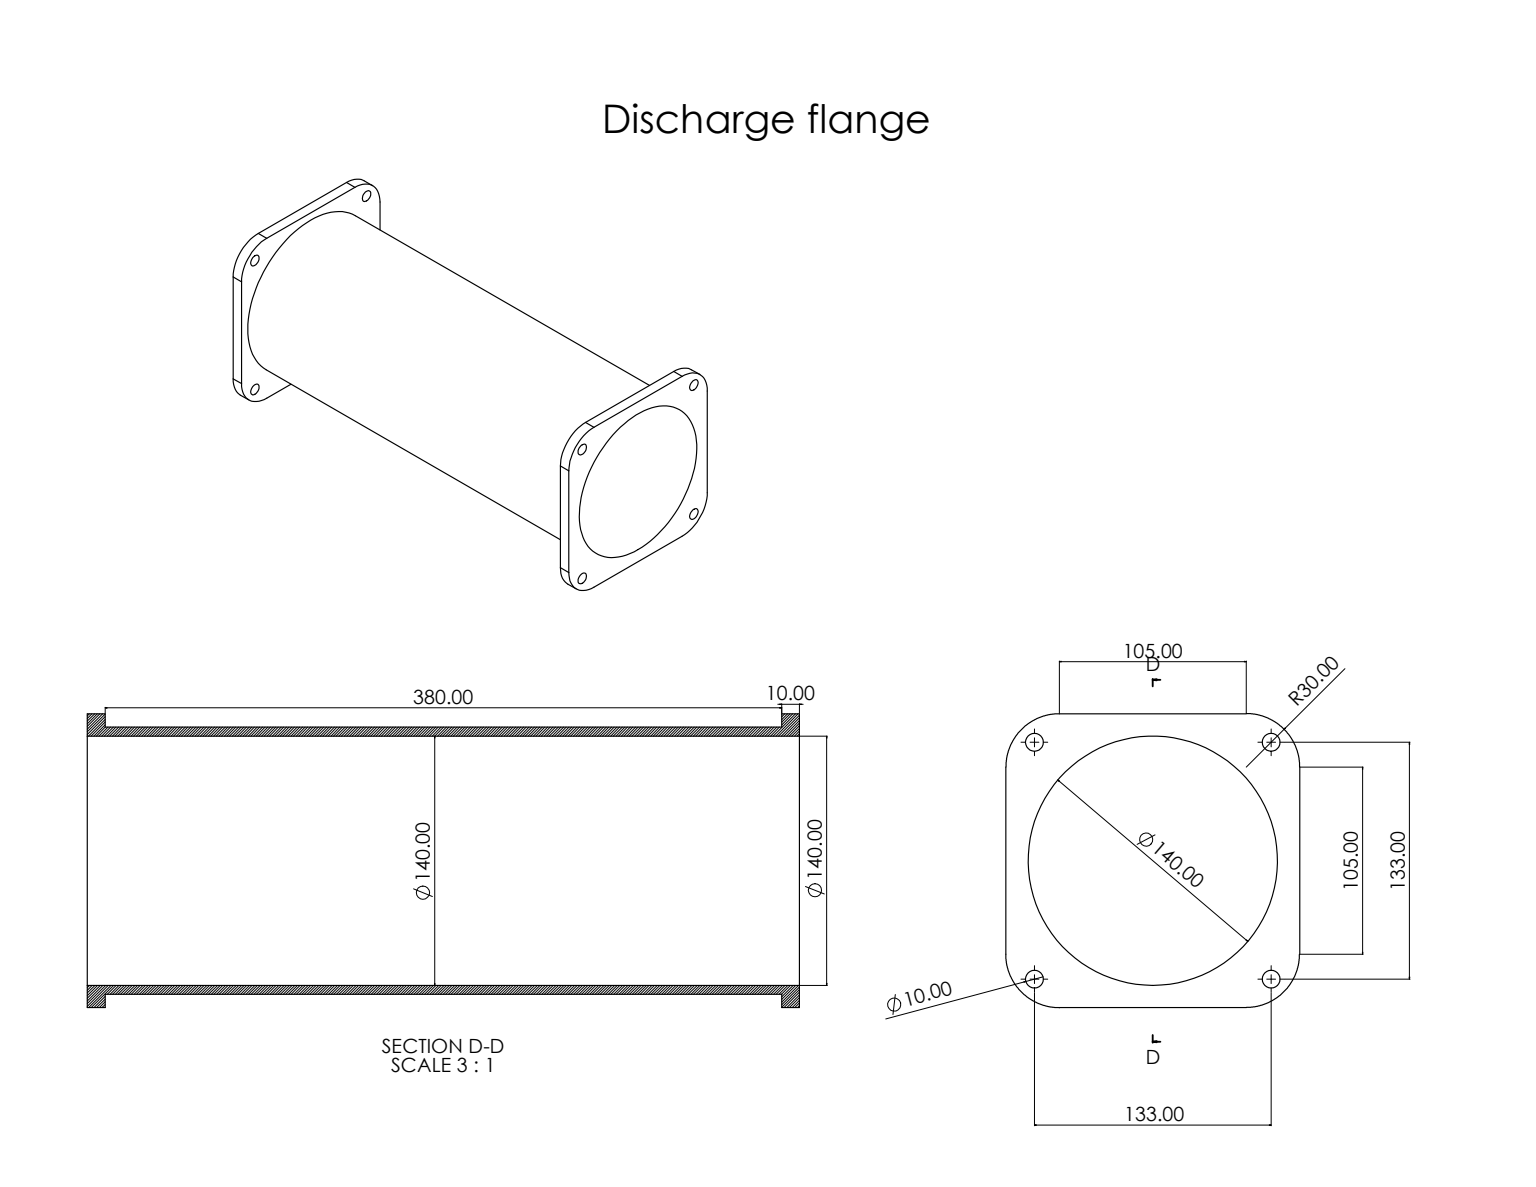
ISO-10303-21;
HEADER;
FILE_DESCRIPTION (('STEP AP214'),
    '1' );
FILE_NAME ('Discharge flange.step',
    '2026-10-27T19:20:31',
    ( '' ),
    ( '' ),
    'SwSTEP 2.0',
    'SolidWorks 2025',
    '' );
FILE_SCHEMA (( 'AUTOMOTIVE_DESIGN' ));
ENDSEC;

DATA;
#22=DIRECTION ( 'NONE',  ( 0.000000000000000000, 0.000000000000000000, 1.000000000000000000 ) ) ;
#32=CARTESIAN_POINT ( 'NONE',  ( -190.0000000000000000, 52.50000000000007816, 52.49999999999999289 ) ) ;
#50=FACE_OUTER_BOUND ( 'NONE', #10007, .T. ) ;
#60=VERTEX_POINT ( 'NONE', #18074 ) ;
#118=ORIENTED_EDGE ( 'NONE', *, *, #8682, .F. ) ;
#155=CARTESIAN_POINT ( 'NONE',  ( 190.0000000000000000, -66.50000000000001421, -66.50000000000005684 ) ) ;
#163=ORIENTED_EDGE ( 'NONE', *, *, #20627, .T. ) ;
#171=CARTESIAN_POINT ( 'NONE',  ( -200.0000000000000000, -66.50000000000001421, -66.50000000000005684 ) ) ;
#193=ADVANCED_FACE ( 'NONE', ( #5707 ), #22219, .T. ) ;
#218=VERTEX_POINT ( 'NONE', #16347 ) ;
#269=DIRECTION ( 'NONE',  ( 0.000000000000000000, -1.000000000000000000, 0.000000000000000000 ) ) ;
#281=ORIENTED_EDGE ( 'NONE', *, *, #13368, .T. ) ;
#283=CARTESIAN_POINT ( 'NONE',  ( -200.0000000000000000, 52.49999999999987210, -82.49999999999998579 ) ) ;
#287=VERTEX_POINT ( 'NONE', #6242 ) ;
#300=ADVANCED_FACE ( 'NONE', ( #8363, #8229, #20751, #2125, #20481, #18473 ), #22483, .F. ) ;
#304=ADVANCED_FACE ( 'NONE', ( #10498 ), #8499, .T. ) ;
#317=DIRECTION ( 'NONE',  ( 1.000000000000000000, -1.836970198721030181E-16, -0.000000000000000000 ) ) ;
#324=DIRECTION ( 'NONE',  ( 1.000000000000000000, 1.836970198721030181E-16, 0.000000000000000000 ) ) ;
#390=ORIENTED_EDGE ( 'NONE', *, *, #13074, .F. ) ;
#407=DIRECTION ( 'NONE',  ( 0.000000000000000000, 0.000000000000000000, 1.000000000000000000 ) ) ;
#423=AXIS2_PLACEMENT_3D ( 'NONE', #16508, #2685, #22769 ) ;
#428=EDGE_LOOP ( 'NONE', ( #390, #21002 ) ) ;
#432=EDGE_LOOP ( 'NONE', ( #11863, #1832, #6303, #14953 ) ) ;
#433=VERTEX_POINT ( 'NONE', #24106 ) ;
#441=FACE_BOUND ( 'NONE', #16176, .T. ) ;
#484=DIRECTION ( 'NONE',  ( -1.000000000000000000, -1.836970198721030181E-16, -0.000000000000000000 ) ) ;
#497=AXIS2_PLACEMENT_3D ( 'NONE', #8550, #23068, #15061 ) ;
#509=VECTOR ( 'NONE', #21184, 1000.000000000000000 ) ;
#531=DIRECTION ( 'NONE',  ( 1.000000000000000000, 1.836970198721030181E-16, -0.000000000000000000 ) ) ;
#555=VERTEX_POINT ( 'NONE', #21999 ) ;
#561=ORIENTED_EDGE ( 'NONE', *, *, #7645, .F. ) ;
#563=ORIENTED_EDGE ( 'NONE', *, *, #7909, .T. ) ;
#600=CARTESIAN_POINT ( 'NONE',  ( -190.0000000000000000, -66.50000000000001421, -66.50000000000005684 ) ) ;
#631=EDGE_CURVE ( 'NONE', #993, #19515, #17493, .T. ) ;
#659=CARTESIAN_POINT ( 'NONE',  ( 190.0000000000000000, 52.50000000000007816, -52.49999999999999289 ) ) ;
#694=AXIS2_PLACEMENT_3D ( 'NONE', #21020, #25155, #15023 ) ;
#727=VECTOR ( 'NONE', #18095, 1000.000000000000000 ) ;
#734=ORIENTED_EDGE ( 'NONE', *, *, #20024, .F. ) ;
#735=ORIENTED_EDGE ( 'NONE', *, *, #6535, .T. ) ;
#737=EDGE_CURVE ( 'NONE', #992, #2989, #22534, .T. ) ;
#820=FACE_OUTER_BOUND ( 'NONE', #17080, .T. ) ;
#845=VECTOR ( 'NONE', #18191, 1000.000000000000000 ) ;
#901=DIRECTION ( 'NONE',  ( 1.000000000000000000, -1.836970198721030181E-16, -0.000000000000000000 ) ) ;
#914=AXIS2_PLACEMENT_3D ( 'NONE', #32, #18248, #10144 ) ;
#948=ORIENTED_EDGE ( 'NONE', *, *, #2831, .T. ) ;
#965=EDGE_CURVE ( 'NONE', #24679, #18072, #13200, .T. ) ;
#971=DIRECTION ( 'NONE',  ( -1.836970198721030181E-16, 1.000000000000000000, 0.000000000000000000 ) ) ;
#992=VERTEX_POINT ( 'NONE', #2965 ) ;
#993=VERTEX_POINT ( 'NONE', #19060 ) ;
#1019=DIRECTION ( 'NONE',  ( -1.000000000000000000, 1.836970198721030181E-16, 0.000000000000000000 ) ) ;
#1053=ADVANCED_FACE ( 'NONE', ( #2269 ), #2400, .T. ) ;
#1066=DIRECTION ( 'NONE',  ( 1.000000000000000000, 1.836970198721030181E-16, 0.000000000000000000 ) ) ;
#1085=CIRCLE ( 'NONE', #21901, 5.000000000000004441 ) ;
#1099=CARTESIAN_POINT ( 'NONE',  ( 199.9999999999999716, 82.50000000000008527, 52.49999999999977973 ) ) ;
#1110=DIRECTION ( 'NONE',  ( 1.000000000000000000, 1.836970198721030181E-16, 0.000000000000000000 ) ) ;
#1112=PRODUCT_DEFINITION ( 'UNKNOWN', '', #12139, #15344 ) ;
#1127=DIRECTION ( 'NONE',  ( -1.000000000000000000, -1.836970198721030181E-16, -0.000000000000000000 ) ) ;
#1134=DIRECTION ( 'NONE',  ( 1.000000000000000000, -1.836970198721030181E-16, -0.000000000000000000 ) ) ;
#1172=CARTESIAN_POINT ( 'NONE',  ( -189.9999999999999716, 82.50000000000008527, -52.49999999999977973 ) ) ;
#1203=FACE_OUTER_BOUND ( 'NONE', #26317, .T. ) ;
#1214=EDGE_LOOP ( 'NONE', ( #19295, #19332, #11818, #2161, #19742, #15932, #25979, #23174 ) ) ;
#1218=DIRECTION ( 'NONE',  ( 1.000000000000000000, 1.836970198721030181E-16, -0.000000000000000000 ) ) ;
#1250=CIRCLE ( 'NONE', #4658, 29.99999999999999289 ) ;
#1303=AXIS2_PLACEMENT_3D ( 'NONE', #1699, #13783, #11796 ) ;
#1313=AXIS2_PLACEMENT_3D ( 'NONE', #15630, #7391, #23754 ) ;
#1318=AXIS2_PLACEMENT_3D ( 'NONE', #22270, #8151, #8412 ) ;
#1321=AXIS2_PLACEMENT_3D ( 'NONE', #15134, #2783, #25005 ) ;
#1364=AXIS2_PLACEMENT_3D ( 'NONE', #13312, #5086, #21558 ) ;
#1370=DIRECTION ( 'NONE',  ( 0.000000000000000000, -1.000000000000000000, 0.000000000000000000 ) ) ;
#1376=ORIENTED_EDGE ( 'NONE', *, *, #13301, .T. ) ;
#1409=DIRECTION ( 'NONE',  ( -1.000000000000000000, 1.836970198721030181E-16, 0.000000000000000000 ) ) ;
#1474=DIRECTION ( 'NONE',  ( 0.000000000000000000, 1.000000000000000000, 0.000000000000000000 ) ) ;
#1482=EDGE_CURVE ( 'NONE', #10703, #20651, #8990, .T. ) ;
#1489=DIRECTION ( 'NONE',  ( 0.000000000000000000, 1.000000000000000000, 0.000000000000000000 ) ) ;
#1497=ORIENTED_EDGE ( 'NONE', *, *, #23863, .F. ) ;
#1520=CARTESIAN_POINT ( 'NONE',  ( -200.0000000000000000, 66.50000000000009948, 66.50000000000005684 ) ) ;
#1577=CARTESIAN_POINT ( 'NONE',  ( 190.0000000000000000, 66.50000000000009948, -66.50000000000005684 ) ) ;
#1589=FACE_OUTER_BOUND ( 'NONE', #24909, .T. ) ;
#1604=CARTESIAN_POINT ( 'NONE',  ( -200.0000000000000000, 0.000000000000000000, 0.000000000000000000 ) ) ;
#1623=ORIENTED_EDGE ( 'NONE', *, *, #25740, .F. ) ;
#1640=EDGE_CURVE ( 'NONE', #23552, #10975, #18053, .T. ) ;
#1669=DIRECTION ( 'NONE',  ( 0.000000000000000000, -1.000000000000000000, 0.000000000000000000 ) ) ;
#1685=FACE_BOUND ( 'NONE', #26345, .T. ) ;
#1699=CARTESIAN_POINT ( 'NONE',  ( -190.0000000000000000, -66.50000000000001421, -66.50000000000005684 ) ) ;
#1701=VECTOR ( 'NONE', #17330, 1000.000000000000000 ) ;
#1725=ORIENTED_EDGE ( 'NONE', *, *, #3774, .F. ) ;
#1728=EDGE_LOOP ( 'NONE', ( #13953, #10765, #25682, #21394 ) ) ;
#1752=LINE ( 'NONE', #26110, #21903 ) ;
#1772=ADVANCED_FACE ( 'NONE', ( #5251 ), #11611, .T. ) ;
#1832=ORIENTED_EDGE ( 'NONE', *, *, #10625, .F. ) ;
#1838=DIRECTION ( 'NONE',  ( 0.000000000000000000, 1.000000000000000000, 0.000000000000000000 ) ) ;
#1851=CARTESIAN_POINT ( 'NONE',  ( 190.0000000000000000, -61.50000000000001421, -66.50000000000005684 ) ) ;
#1866=ORIENTED_EDGE ( 'NONE', *, *, #7645, .T. ) ;
#1888=VERTEX_POINT ( 'NONE', #25639 ) ;
#1934=AXIS2_PLACEMENT_3D ( 'NONE', #1520, #11748, #11232 ) ;
#1964=AXIS2_PLACEMENT_3D ( 'NONE', #11885, #17999, #22143 ) ;
#1971=DIRECTION ( 'NONE',  ( 1.000000000000000000, 1.836970198721030181E-16, 0.000000000000000000 ) ) ;
#1982=LINE ( 'NONE', #3983, #845 ) ;
#2006=ADVANCED_FACE ( 'NONE', ( #3029 ), #5031, .F. ) ;
#2014=EDGE_CURVE ( 'NONE', #6828, #18680, #13381, .T. ) ;
#2056=APPLICATION_CONTEXT ( 'automotive_design' ) ;
#2120=EDGE_LOOP ( 'NONE', ( #10499, #15535, #8500, #5942 ) ) ;
#2125=FACE_BOUND ( 'NONE', #428, .T. ) ;
#2129=DIRECTION ( 'NONE',  ( 1.000000000000000000, -1.836970198721030181E-16, -0.000000000000000000 ) ) ;
#2161=ORIENTED_EDGE ( 'NONE', *, *, #13851, .F. ) ;
#2166=EDGE_LOOP ( 'NONE', ( #25011, #25719, #18779, #2522 ) ) ;
#2178=CARTESIAN_POINT ( 'NONE',  ( -190.0000000000000000, 66.50000000000009948, 66.50000000000005684 ) ) ;
#2240=EDGE_CURVE ( 'NONE', #218, #23932, #5326, .T. ) ;
#2249=CARTESIAN_POINT ( 'NONE',  ( -190.0000000000000000, -52.49999999999992895, -52.49999999999999289 ) ) ;
#2255=DIRECTION ( 'NONE',  ( 1.836970198721030181E-16, 1.000000000000000000, 0.000000000000000000 ) ) ;
#2256=EDGE_CURVE ( 'NONE', #18680, #16217, #11268, .T. ) ;
#2269=FACE_OUTER_BOUND ( 'NONE', #1728, .T. ) ;
#2277=LINE ( 'NONE', #10386, #3682 ) ;
#2287=EDGE_LOOP ( 'NONE', ( #15332, #4523, #9187, #4693 ) ) ;
#2321=ORIENTED_EDGE ( 'NONE', *, *, #26327, .F. ) ;
#2352=AXIS2_PLACEMENT_3D ( 'NONE', #13008, #11378, #25253 ) ;
#2362=CARTESIAN_POINT ( 'NONE',  ( 200.0000000000000000, 75.00000000000000000, 0.000000000000000000 ) ) ;
#2379=VECTOR ( 'NONE', #1409, 1000.000000000000000 ) ;
#2384=VERTEX_POINT ( 'NONE', #18806 ) ;
#2400=CYLINDRICAL_SURFACE ( 'NONE', #15990, 29.99999999999999289 ) ;
#2415=CARTESIAN_POINT ( 'NONE',  ( -190.0000000000000000, 52.50000000000007816, -52.49999999999999289 ) ) ;
#2421=ORIENTED_EDGE ( 'NONE', *, *, #965, .T. ) ;
#2468=CARTESIAN_POINT ( 'NONE',  ( -190.0000000000000000, 71.50000000000009948, 66.50000000000005684 ) ) ;
#2487=DIRECTION ( 'NONE',  ( 0.000000000000000000, 1.000000000000000000, 0.000000000000000000 ) ) ;
#2489=CARTESIAN_POINT ( 'NONE',  ( 200.0000000000000000, -66.50000000000001421, 66.50000000000005684 ) ) ;
#2495=DIRECTION ( 'NONE',  ( -1.000000000000000000, 1.836970198721030181E-16, 0.000000000000000000 ) ) ;
#2522=ORIENTED_EDGE ( 'NONE', *, *, #3703, .F. ) ;
#2550=CYLINDRICAL_SURFACE ( 'NONE', #10885, 5.000000000000004441 ) ;
#2557=ORIENTED_EDGE ( 'NONE', *, *, #2240, .T. ) ;
#2562=CARTESIAN_POINT ( 'NONE',  ( 190.0000000000000284, -82.49999999999990052, 52.49999999999977973 ) ) ;
#2593=ORIENTED_EDGE ( 'NONE', *, *, #19566, .F. ) ;
#2636=LINE ( 'NONE', #24852, #7070 ) ;
#2643=AXIS2_PLACEMENT_3D ( 'NONE', #10104, #24350, #6114 ) ;
#2655=ORIENTED_EDGE ( 'NONE', *, *, #24117, .T. ) ;
#2672=EDGE_CURVE ( 'NONE', #17972, #19937, #22628, .T. ) ;
#2673=CARTESIAN_POINT ( 'NONE',  ( -200.0000000000000284, -82.49999999999991473, -52.49999999999977973 ) ) ;
#2684=CYLINDRICAL_SURFACE ( 'NONE', #19005, 5.000000000000004441 ) ;
#2685=DIRECTION ( 'NONE',  ( 1.000000000000000000, 1.836970198721030181E-16, -0.000000000000000000 ) ) ;
#2727=ORIENTED_EDGE ( 'NONE', *, *, #19780, .T. ) ;
#2730=CARTESIAN_POINT ( 'NONE',  ( -200.0000000000000000, -61.50000000000001421, 66.50000000000005684 ) ) ;
#2735=DIRECTION ( 'NONE',  ( 0.000000000000000000, -1.000000000000000000, 0.000000000000000000 ) ) ;
#2760=VERTEX_POINT ( 'NONE', #2673 ) ;
#2783=DIRECTION ( 'NONE',  ( -1.000000000000000000, 1.836970198721030181E-16, 0.000000000000000000 ) ) ;
#2792=EDGE_CURVE ( 'NONE', #4564, #9028, #14622, .T. ) ;
#2831=EDGE_CURVE ( 'NONE', #18337, #9825, #12145, .T. ) ;
#2841=EDGE_CURVE ( 'NONE', #7865, #20847, #25329, .T. ) ;
#2892=LINE ( 'NONE', #15368, #5991 ) ;
#2923=CARTESIAN_POINT ( 'NONE',  ( 190.0000000000000000, 71.50000000000009948, 66.50000000000005684 ) ) ;
#2965=CARTESIAN_POINT ( 'NONE',  ( 190.0000000000000000, -71.50000000000002842, -66.50000000000005684 ) ) ;
#2989=VERTEX_POINT ( 'NONE', #5300 ) ;
#3029=FACE_OUTER_BOUND ( 'NONE', #3584, .T. ) ;
#3036=DIRECTION ( 'NONE',  ( 0.000000000000000000, 0.000000000000000000, 1.000000000000000000 ) ) ;
#3079=ORIENTED_EDGE ( 'NONE', *, *, #23863, .T. ) ;
#3082=CARTESIAN_POINT ( 'NONE',  ( 200.0000000000000000, -69.99999999999985789, 0.000000000000000000 ) ) ;
#3085=EDGE_LOOP ( 'NONE', ( #20124, #5286, #15365, #2593 ) ) ;
#3097=CARTESIAN_POINT ( 'NONE',  ( -200.0000000000000000, 71.50000000000009948, -66.50000000000005684 ) ) ;
#3100=DIRECTION ( 'NONE',  ( 0.000000000000000000, 1.000000000000000000, 0.000000000000000000 ) ) ;
#3139=VERTEX_POINT ( 'NONE', #12045 ) ;
#3145=CARTESIAN_POINT ( 'NONE',  ( 200.0000000000000284, -82.49999999999991473, -52.49999999999977973 ) ) ;
#3210=DIRECTION ( 'NONE',  ( 1.000000000000000000, 1.836970198721030181E-16, 0.000000000000000000 ) ) ;
#3270=CARTESIAN_POINT ( 'NONE',  ( -190.0000000000000000, 61.50000000000009948, -66.50000000000005684 ) ) ;
#3271=CARTESIAN_POINT ( 'NONE',  ( 190.0000000000000000, -71.50000000000002842, 66.50000000000005684 ) ) ;
#3272=CIRCLE ( 'NONE', #18137, 5.000000000000004441 ) ;
#3319=PLANE ( 'NONE',  #14956 ) ;
#3326=ORIENTED_EDGE ( 'NONE', *, *, #14182, .T. ) ;
#3367=CARTESIAN_POINT ( 'NONE',  ( -190.0000000000000000, -74.99999999999995737, 0.000000000000000000 ) ) ;
#3373=DIRECTION ( 'NONE',  ( 1.000000000000000000, -1.836970198721030181E-16, 0.000000000000000000 ) ) ;
#3443=PLANE ( 'NONE',  #15673 ) ;
#3446=VERTEX_POINT ( 'NONE', #7334 ) ;
#3458=EDGE_LOOP ( 'NONE', ( #25215, #16114, #9669, #11794 ) ) ;
#3467=CARTESIAN_POINT ( 'NONE',  ( -189.9999999999999716, 82.50000000000008527, -52.49999999999977973 ) ) ;
#3522=CYLINDRICAL_SURFACE ( 'NONE', #17630, 5.000000000000004441 ) ;
#3532=EDGE_CURVE ( 'NONE', #21182, #3446, #21578, .T. ) ;
#3546=ORIENTED_EDGE ( 'NONE', *, *, #19780, .F. ) ;
#3584=EDGE_LOOP ( 'NONE', ( #7054, #10530, #26087, #25050 ) ) ;
#3588=DIRECTION ( 'NONE',  ( -1.000000000000000000, -1.836970198721030181E-16, -0.000000000000000000 ) ) ;
#3611=EDGE_CURVE ( 'NONE', #16217, #18680, #15942, .T. ) ;
#3616=AXIS2_PLACEMENT_3D ( 'NONE', #19733, #23355, #5132 ) ;
#3680=ORIENTED_EDGE ( 'NONE', *, *, #8682, .T. ) ;
#3682=VECTOR ( 'NONE', #18497, 1000.000000000000000 ) ;
#3689=EDGE_CURVE ( 'NONE', #10975, #23552, #25752, .T. ) ;
#3703=EDGE_CURVE ( 'NONE', #8862, #19485, #1752, .T. ) ;
#3772=FACE_OUTER_BOUND ( 'NONE', #17773, .T. ) ;
#3774=EDGE_CURVE ( 'NONE', #433, #4824, #19279, .T. ) ;
#3792=AXIS2_PLACEMENT_3D ( 'NONE', #2489, #4365, #14585 ) ;
#3797=DIRECTION ( 'NONE',  ( -1.000000000000000000, -1.836970198721030181E-16, -0.000000000000000000 ) ) ;
#3824=CARTESIAN_POINT ( 'NONE',  ( 190.0000000000000000, 66.50000000000009948, 66.50000000000005684 ) ) ;
#3862=EDGE_CURVE ( 'NONE', #19937, #8803, #7875, .T. ) ;
#3886=VECTOR ( 'NONE', #1019, 1000.000000000000000 ) ;
#3890=LINE ( 'NONE', #8129, #4264 ) ;
#3892=LINE ( 'NONE', #5738, #13231 ) ;
#3903=ORIENTED_EDGE ( 'NONE', *, *, #22166, .F. ) ;
#3934=AXIS2_PLACEMENT_3D ( 'NONE', #26310, #8318, #10455 ) ;
#3964=EDGE_LOOP ( 'NONE', ( #23997, #7152, #21523, #24412 ) ) ;
#3968=ADVANCED_FACE ( 'NONE', ( #25902 ), #20039, .T. ) ;
#3972=CYLINDRICAL_SURFACE ( 'NONE', #11313, 5.000000000000004441 ) ;
#3983=CARTESIAN_POINT ( 'NONE',  ( -190.0000000000000000, 82.50000000000008527, 52.49999999999979394 ) ) ;
#3990=ORIENTED_EDGE ( 'NONE', *, *, #7909, .F. ) ;
#4020=DIRECTION ( 'NONE',  ( -1.000000000000000000, 1.836970198721030181E-16, 0.000000000000000000 ) ) ;
#4026=DIRECTION ( 'NONE',  ( 1.000000000000000000, 1.836970198721030181E-16, 0.000000000000000000 ) ) ;
#4028=( LENGTH_UNIT ( ) NAMED_UNIT ( * ) SI_UNIT ( .MILLI., .METRE. ) );
#4043=CARTESIAN_POINT ( 'NONE',  ( -190.0000000000000000, 52.49999999999987210, -82.49999999999998579 ) ) ;
#4055=PLANE ( 'NONE',  #1964 ) ;
#4071=CARTESIAN_POINT ( 'NONE',  ( 200.0000000000000000, 52.50000000000007816, 52.49999999999999289 ) ) ;
#4140=VECTOR ( 'NONE', #16370, 1000.000000000000000 ) ;
#4200=ORIENTED_EDGE ( 'NONE', *, *, #9474, .F. ) ;
#4222=AXIS2_PLACEMENT_3D ( 'NONE', #23852, #25868, #5503 ) ;
#4223=ADVANCED_FACE ( 'NONE', ( #50 ), #4055, .T. ) ;
#4233=ORIENTED_EDGE ( 'NONE', *, *, #3689, .F. ) ;
#4262=DIRECTION ( 'NONE',  ( -1.000000000000000000, 1.836970198721030181E-16, 0.000000000000000000 ) ) ;
#4264=VECTOR ( 'NONE', #9995, 1000.000000000000000 ) ;
#4288=CARTESIAN_POINT ( 'NONE',  ( -190.0000000000000000, -52.49999999999970868, 82.49999999999998579 ) ) ;
#4302=DIRECTION ( 'NONE',  ( -0.000000000000000000, -0.000000000000000000, 1.000000000000000000 ) ) ;
#4365=DIRECTION ( 'NONE',  ( 1.000000000000000000, 1.836970198721030181E-16, -0.000000000000000000 ) ) ;
#4385=ORIENTED_EDGE ( 'NONE', *, *, #6535, .F. ) ;
#4446=DIRECTION ( 'NONE',  ( 0.000000000000000000, -1.000000000000000000, 0.000000000000000000 ) ) ;
#4468=CARTESIAN_POINT ( 'NONE',  ( 200.0000000000000000, -61.50000000000001421, 66.50000000000005684 ) ) ;
#4501=VECTOR ( 'NONE', #17086, 1000.000000000000000 ) ;
#4502=AXIS2_PLACEMENT_3D ( 'NONE', #5106, #5352, #13211 ) ;
#4520=EDGE_CURVE ( 'NONE', #2760, #1888, #11698, .T. ) ;
#4523=ORIENTED_EDGE ( 'NONE', *, *, #2841, .T. ) ;
#4529=DIRECTION ( 'NONE',  ( 0.000000000000000000, -1.000000000000000000, 0.000000000000000000 ) ) ;
#4564=VERTEX_POINT ( 'NONE', #21957 ) ;
#4576=CARTESIAN_POINT ( 'NONE',  ( 190.0000000000000000, 52.50000000000007816, 52.49999999999999289 ) ) ;
#4594=ORIENTED_EDGE ( 'NONE', *, *, #19220, .T. ) ;
#4605=CARTESIAN_POINT ( 'NONE',  ( -190.0000000000000000, -52.49999999999972289, -82.49999999999998579 ) ) ;
#4632=DIRECTION ( 'NONE',  ( 1.000000000000000000, 1.836970198721030181E-16, 0.000000000000000000 ) ) ;
#4647=CARTESIAN_POINT ( 'NONE',  ( 190.0000000000000284, -82.49999999999990052, 52.49999999999977973 ) ) ;
#4657=CARTESIAN_POINT ( 'NONE',  ( 200.0000000000000000, 66.50000000000009948, -66.50000000000005684 ) ) ;
#4658=AXIS2_PLACEMENT_3D ( 'NONE', #13819, #1218, #15681 ) ;
#4679=EDGE_LOOP ( 'NONE', ( #25946, #11681, #735, #14353 ) ) ;
#4693=ORIENTED_EDGE ( 'NONE', *, *, #19719, .F. ) ;
#4694=ORIENTED_EDGE ( 'NONE', *, *, #1482, .T. ) ;
#4702=EDGE_CURVE ( 'NONE', #23932, #17972, #15684, .T. ) ;
#4731=DIRECTION ( 'NONE',  ( 0.000000000000000000, -1.000000000000000000, 0.000000000000000000 ) ) ;
#4791=VERTEX_POINT ( 'NONE', #5718 ) ;
#4824=VERTEX_POINT ( 'NONE', #13823 ) ;
#4827=EDGE_LOOP ( 'NONE', ( #14187, #10973 ) ) ;
#4857=ORIENTED_EDGE ( 'NONE', *, *, #25450, .F. ) ;
#4863=AXIS2_PLACEMENT_3D ( 'NONE', #3824, #17770, #17904 ) ;
#4895=DIRECTION ( 'NONE',  ( 1.000000000000000000, 1.836970198721030181E-16, 0.000000000000000000 ) ) ;
#4958=ORIENTED_EDGE ( 'NONE', *, *, #2792, .F. ) ;
#4961=CIRCLE ( 'NONE', #9195, 5.000000000000004441 ) ;
#4966=DIRECTION ( 'NONE',  ( 0.000000000000000000, -1.000000000000000000, 0.000000000000000000 ) ) ;
#4970=AXIS2_PLACEMENT_3D ( 'NONE', #10637, #4262, #2255 ) ;
#4971=DIRECTION ( 'NONE',  ( 1.000000000000000000, 1.836970198721030181E-16, 0.000000000000000000 ) ) ;
#4995=DIRECTION ( 'NONE',  ( 0.000000000000000000, -1.000000000000000000, 0.000000000000000000 ) ) ;
#5026=DIRECTION ( 'NONE',  ( 0.000000000000000000, -1.000000000000000000, 0.000000000000000000 ) ) ;
#5031=PLANE ( 'NONE',  #2352 ) ;
#5050=VECTOR ( 'NONE', #7667, 1000.000000000000000 ) ;
#5075=EDGE_CURVE ( 'NONE', #218, #24643, #19992, .T. ) ;
#5086=DIRECTION ( 'NONE',  ( -1.000000000000000000, 1.836970198721030181E-16, 0.000000000000000000 ) ) ;
#5092=FACE_BOUND ( 'NONE', #7433, .T. ) ;
#5106=CARTESIAN_POINT ( 'NONE',  ( -200.0000000000000000, -66.50000000000001421, 66.50000000000005684 ) ) ;
#5109=DIRECTION ( 'NONE',  ( 0.000000000000000000, 1.000000000000000000, 0.000000000000000000 ) ) ;
#5132=DIRECTION ( 'NONE',  ( 0.000000000000000000, 1.000000000000000000, 0.000000000000000000 ) ) ;
#5165=AXIS2_PLACEMENT_3D ( 'NONE', #9690, #7952, #17796 ) ;
#5193=CYLINDRICAL_SURFACE ( 'NONE', #10940, 5.000000000000004441 ) ;
#5221=DIRECTION ( 'NONE',  ( 0.000000000000000000, -1.000000000000000000, 0.000000000000000000 ) ) ;
#5251=FACE_OUTER_BOUND ( 'NONE', #6274, .T. ) ;
#5254=EDGE_CURVE ( 'NONE', #19106, #9028, #7453, .T. ) ;
#5283=LINE ( 'NONE', #19507, #23365 ) ;
#5286=ORIENTED_EDGE ( 'NONE', *, *, #2014, .T. ) ;
#5300=CARTESIAN_POINT ( 'NONE',  ( 200.0000000000000000, -71.50000000000002842, -66.50000000000005684 ) ) ;
#5325=AXIS2_PLACEMENT_3D ( 'NONE', #600, #19337, #4995 ) ;
#5326=CIRCLE ( 'NONE', #24003, 30.00000000000000355 ) ;
#5352=DIRECTION ( 'NONE',  ( 1.000000000000000000, -1.836970198721030181E-16, -0.000000000000000000 ) ) ;
#5367=CARTESIAN_POINT ( 'NONE',  ( -200.0000000000000000, 52.49999999999987210, 82.49999999999998579 ) ) ;
#5390=EDGE_CURVE ( 'NONE', #7865, #22425, #6002, .T. ) ;
#5459=DIRECTION ( 'NONE',  ( 1.000000000000000000, -1.836970198721030181E-16, -0.000000000000000000 ) ) ;
#5488=VERTEX_POINT ( 'NONE', #7841 ) ;
#5495=CIRCLE ( 'NONE', #23752, 5.000000000000004441 ) ;
#5500=CYLINDRICAL_SURFACE ( 'NONE', #23652, 30.00000000000000711 ) ;
#5503=DIRECTION ( 'NONE',  ( 0.000000000000000000, -1.000000000000000000, 0.000000000000000000 ) ) ;
#5552=UNCERTAINTY_MEASURE_WITH_UNIT (LENGTH_MEASURE( 1.000000000000000082E-05 ), #5889, 'distance_accuracy_value', 'NONE');
#5574=DIRECTION ( 'NONE',  ( 1.000000000000000000, 1.836970198721030181E-16, 0.000000000000000000 ) ) ;
#5600=DIRECTION ( 'NONE',  ( 1.000000000000000000, 1.836970198721030181E-16, -0.000000000000000000 ) ) ;
#5604=CIRCLE ( 'NONE', #10729, 69.99999999999992895 ) ;
#5642=ORIENTED_EDGE ( 'NONE', *, *, #23903, .T. ) ;
#5664=FACE_OUTER_BOUND ( 'NONE', #8219, .T. ) ;
#5707=FACE_OUTER_BOUND ( 'NONE', #4679, .T. ) ;
#5718=CARTESIAN_POINT ( 'NONE',  ( -190.0000000000000284, -82.49999999999991473, -52.49999999999977973 ) ) ;
#5719=EDGE_CURVE ( 'NONE', #21182, #22119, #21953, .T. ) ;
#5720=ADVANCED_FACE ( 'NONE', ( #14161 ), #18148, .T. ) ;
#5738=CARTESIAN_POINT ( 'NONE',  ( -190.0000000000000000, -71.50000000000002842, 66.50000000000005684 ) ) ;
#5747=EDGE_LOOP ( 'NONE', ( #1376, #23519, #3680, #15738, #16613, #24918, #22384, #22123 ) ) ;
#5748=EDGE_LOOP ( 'NONE', ( #7100, #1497 ) ) ;
#5758=CIRCLE ( 'NONE', #15941, 30.00000000000000355 ) ;
#5774=VECTOR ( 'NONE', #11426, 1000.000000000000000 ) ;
#5871=ORIENTED_EDGE ( 'NONE', *, *, #15011, .F. ) ;
#5884=ORIENTED_EDGE ( 'NONE', *, *, #9469, .F. ) ;
#5889=( LENGTH_UNIT ( ) NAMED_UNIT ( * ) SI_UNIT ( .MILLI., .METRE. ) );
#5895=CARTESIAN_POINT ( 'NONE',  ( 190.0000000000000000, -52.49999999999970868, 82.49999999999998579 ) ) ;
#5912=ADVANCED_FACE ( 'NONE', ( #25747 ), #9499, .F. ) ;
#5942=ORIENTED_EDGE ( 'NONE', *, *, #15794, .F. ) ;
#5952=AXIS2_PLACEMENT_3D ( 'NONE', #155, #4026, #18376 ) ;
#5991=VECTOR ( 'NONE', #15108, 1000.000000000000000 ) ;
#6002=LINE ( 'NONE', #17956, #727 ) ;
#6021=CIRCLE ( 'NONE', #497, 29.99999999999999645 ) ;
#6058=FACE_OUTER_BOUND ( 'NONE', #432, .T. ) ;
#6089=PLANE ( 'NONE',  #12589 ) ;
#6114=DIRECTION ( 'NONE',  ( 0.000000000000000000, -1.000000000000000000, 0.000000000000000000 ) ) ;
#6152=CYLINDRICAL_SURFACE ( 'NONE', #914, 30.00000000000000355 ) ;
#6156=EDGE_CURVE ( 'NONE', #8862, #24345, #15958, .T. ) ;
#6225=VECTOR ( 'NONE', #20829, 1000.000000000000000 ) ;
#6242=CARTESIAN_POINT ( 'NONE',  ( -190.0000000000000000, -71.50000000000002842, 66.50000000000005684 ) ) ;
#6245=LINE ( 'NONE', #14358, #17485 ) ;
#6255=CARTESIAN_POINT ( 'NONE',  ( -190.0000000000000000, -52.49999999999992895, -52.49999999999999289 ) ) ;
#6274=EDGE_LOOP ( 'NONE', ( #21808, #4958, #19084, #13556 ) ) ;
#6278=EDGE_LOOP ( 'NONE', ( #11152, #13148 ) ) ;
#6303=ORIENTED_EDGE ( 'NONE', *, *, #15250, .T. ) ;
#6305=VERTEX_POINT ( 'NONE', #13685 ) ;
#6379=DIRECTION ( 'NONE',  ( -1.000000000000000000, 1.836970198721030181E-16, 0.000000000000000000 ) ) ;
#6380=EDGE_CURVE ( 'NONE', #5488, #4791, #9064, .T. ) ;
#6393=VERTEX_POINT ( 'NONE', #3082 ) ;
#6423=CARTESIAN_POINT ( 'NONE',  ( -200.0000000000000000, -66.50000000000001421, -66.50000000000005684 ) ) ;
#6435=ORIENTED_EDGE ( 'NONE', *, *, #6869, .T. ) ;
#6535=EDGE_CURVE ( 'NONE', #7186, #4564, #11147, .T. ) ;
#6541=EDGE_CURVE ( 'NONE', #9825, #18337, #18740, .T. ) ;
#6604=DIRECTION ( 'NONE',  ( 0.000000000000000000, 1.000000000000000000, 0.000000000000000000 ) ) ;
#6626=AXIS2_PLACEMENT_3D ( 'NONE', #14781, #13060, #22649 ) ;
#6631=DIRECTION ( 'NONE',  ( -1.000000000000000000, 1.836970198721030181E-16, 0.000000000000000000 ) ) ;
#6662=DIRECTION ( 'NONE',  ( 0.000000000000000000, -1.000000000000000000, 0.000000000000000000 ) ) ;
#6668=ORIENTED_EDGE ( 'NONE', *, *, #5390, .T. ) ;
#6682=LINE ( 'NONE', #18932, #9406 ) ;
#6701=ORIENTED_EDGE ( 'NONE', *, *, #14853, .F. ) ;
#6741=CYLINDRICAL_SURFACE ( 'NONE', #10700, 5.000000000000004441 ) ;
#6742=CYLINDRICAL_SURFACE ( 'NONE', #24945, 5.000000000000004441 ) ;
#6756=DIRECTION ( 'NONE',  ( 1.000000000000000000, -1.836970198721030181E-16, -0.000000000000000000 ) ) ;
#6794=AXIS2_PLACEMENT_3D ( 'NONE', #19130, #6756, #13017 ) ;
#6828=VERTEX_POINT ( 'NONE', #26217 ) ;
#6842=AXIS2_PLACEMENT_3D ( 'NONE', #9932, #8063, #18038 ) ;
#6844=VECTOR ( 'NONE', #7582, 1000.000000000000000 ) ;
#6850=DIRECTION ( 'NONE',  ( 0.000000000000000000, 1.000000000000000000, 0.000000000000000000 ) ) ;
#6869=EDGE_CURVE ( 'NONE', #4791, #6305, #9382, .T. ) ;
#6965=VERTEX_POINT ( 'NONE', #12753 ) ;
#6968=CARTESIAN_POINT ( 'NONE',  ( -190.0000000000000000, 66.50000000000009948, -66.50000000000005684 ) ) ;
#6994=LINE ( 'NONE', #3270, #20804 ) ;
#7030=VECTOR ( 'NONE', #407, 1000.000000000000000 ) ;
#7054=ORIENTED_EDGE ( 'NONE', *, *, #11709, .T. ) ;
#7067=ORIENTED_EDGE ( 'NONE', *, *, #9474, .T. ) ;
#7070=VECTOR ( 'NONE', #13004, 1000.000000000000000 ) ;
#7089=CARTESIAN_POINT ( 'NONE',  ( 190.0000000000000000, 61.50000000000009948, 66.50000000000005684 ) ) ;
#7092=DIRECTION ( 'NONE',  ( -1.000000000000000000, 1.836970198721030181E-16, 0.000000000000000000 ) ) ;
#7100=ORIENTED_EDGE ( 'NONE', *, *, #7510, .F. ) ;
#7152=ORIENTED_EDGE ( 'NONE', *, *, #15011, .T. ) ;
#7180=VERTEX_POINT ( 'NONE', #9148 ) ;
#7185=EDGE_CURVE ( 'NONE', #20651, #23802, #19910, .T. ) ;
#7186=VERTEX_POINT ( 'NONE', #11790 ) ;
#7194=ADVANCED_FACE ( 'NONE', ( #17636 ), #9799, .F. ) ;
#7215=CARTESIAN_POINT ( 'NONE',  ( -190.0000000000000000, -52.49999999999970868, 82.49999999999998579 ) ) ;
#7222=CIRCLE ( 'NONE', #14018, 5.000000000000004441 ) ;
#7233=CARTESIAN_POINT ( 'NONE',  ( 200.0000000000000000, -71.50000000000002842, 66.50000000000005684 ) ) ;
#7307=ORIENTED_EDGE ( 'NONE', *, *, #23949, .F. ) ;
#7319=LINE ( 'NONE', #9579, #21198 ) ;
#7334=CARTESIAN_POINT ( 'NONE',  ( 200.0000000000000000, 61.50000000000009948, 66.50000000000005684 ) ) ;
#7338=CARTESIAN_POINT ( 'NONE',  ( 190.0000000000000000, 66.50000000000009948, 66.50000000000005684 ) ) ;
#7391=DIRECTION ( 'NONE',  ( 1.000000000000000000, 1.836970198721030181E-16, 0.000000000000000000 ) ) ;
#7406=EDGE_CURVE ( 'NONE', #24210, #8803, #18472, .T. ) ;
#7428=( GEOMETRIC_REPRESENTATION_CONTEXT ( 3 ) GLOBAL_UNCERTAINTY_ASSIGNED_CONTEXT ( ( #15650 ) ) GLOBAL_UNIT_ASSIGNED_CONTEXT ( ( #4028, #14250, #22518 ) ) REPRESENTATION_CONTEXT ( 'NONE', 'WORKASPACE' ) );
#7429=ORIENTED_EDGE ( 'NONE', *, *, #13444, .F. ) ;
#7433=EDGE_LOOP ( 'NONE', ( #10400, #16251 ) ) ;
#7439=CARTESIAN_POINT ( 'NONE',  ( -200.0000000000000000, 66.50000000000009948, -66.50000000000005684 ) ) ;
#7453=LINE ( 'NONE', #11445, #23211 ) ;
#7458=AXIS2_PLACEMENT_3D ( 'NONE', #15240, #11765, #15875 ) ;
#7470=AXIS2_PLACEMENT_3D ( 'NONE', #20459, #901, #6604 ) ;
#7477=CARTESIAN_POINT ( 'NONE',  ( -200.0000000000000000, 0.000000000000000000, 0.000000000000000000 ) ) ;
#7485=AXIS2_PLACEMENT_3D ( 'NONE', #24288, #20025, #19885 ) ;
#7510=EDGE_CURVE ( 'NONE', #287, #6828, #3272, .T. ) ;
#7541=CARTESIAN_POINT ( 'NONE',  ( -190.0000000000000000, 66.50000000000009948, -66.50000000000005684 ) ) ;
#7551=ORIENTED_EDGE ( 'NONE', *, *, #10708, .T. ) ;
#7582=DIRECTION ( 'NONE',  ( -0.000000000000000000, -0.000000000000000000, 1.000000000000000000 ) ) ;
#7604=DIRECTION ( 'NONE',  ( 0.000000000000000000, -1.000000000000000000, 0.000000000000000000 ) ) ;
#7645=EDGE_CURVE ( 'NONE', #11213, #10975, #9532, .T. ) ;
#7659=EDGE_LOOP ( 'NONE', ( #25111, #14780, #18300, #18336 ) ) ;
#7667=DIRECTION ( 'NONE',  ( -1.000000000000000000, -1.836970198721030181E-16, -0.000000000000000000 ) ) ;
#7692=EDGE_LOOP ( 'NONE', ( #19581, #18546, #11366, #9730 ) ) ;
#7726=ORIENTED_EDGE ( 'NONE', *, *, #9144, .T. ) ;
#7738=DIRECTION ( 'NONE',  ( -1.000000000000000000, 1.836970198721030181E-16, 0.000000000000000000 ) ) ;
#7750=EDGE_CURVE ( 'NONE', #14209, #23802, #14456, .T. ) ;
#7841=CARTESIAN_POINT ( 'NONE',  ( -190.0000000000000284, -82.49999999999990052, 52.49999999999977973 ) ) ;
#7865=VERTEX_POINT ( 'NONE', #17486 ) ;
#7875=CIRCLE ( 'NONE', #26183, 30.00000000000000355 ) ;
#7898=DIRECTION ( 'NONE',  ( -1.000000000000000000, -1.836970198721030181E-16, -0.000000000000000000 ) ) ;
#7904=DIRECTION ( 'NONE',  ( 1.000000000000000000, 1.836970198721030181E-16, 0.000000000000000000 ) ) ;
#7909=EDGE_CURVE ( 'NONE', #17301, #6965, #2892, .T. ) ;
#7937=CARTESIAN_POINT ( 'NONE',  ( 190.0000000000000000, 71.50000000000009948, -66.50000000000005684 ) ) ;
#7952=DIRECTION ( 'NONE',  ( 1.000000000000000000, -1.836970198721030181E-16, -0.000000000000000000 ) ) ;
#7954=SHAPE_DEFINITION_REPRESENTATION ( #23973, #12169 ) ;
#7994=CARTESIAN_POINT ( 'NONE',  ( 0.000000000000000000, 0.000000000000000000, 0.000000000000000000 ) ) ;
#8006=EDGE_CURVE ( 'NONE', #22119, #2384, #14846, .T. ) ;
#8037=CARTESIAN_POINT ( 'NONE',  ( -200.0000000000000000, 0.000000000000000000, 0.000000000000000000 ) ) ;
#8054=CIRCLE ( 'NONE', #423, 5.000000000000004441 ) ;
#8063=DIRECTION ( 'NONE',  ( 1.000000000000000000, 1.836970198721030181E-16, 0.000000000000000000 ) ) ;
#8086=ORIENTED_EDGE ( 'NONE', *, *, #24913, .T. ) ;
#8129=CARTESIAN_POINT ( 'NONE',  ( 190.0000000000000000, -52.49999999999970868, 82.49999999999998579 ) ) ;
#8130=DIRECTION ( 'NONE',  ( -1.000000000000000000, 1.836970198721030181E-16, 0.000000000000000000 ) ) ;
#8144=( NAMED_UNIT ( * ) PLANE_ANGLE_UNIT ( ) SI_UNIT ( $, .RADIAN. ) );
#8145=EDGE_CURVE ( 'NONE', #4791, #2760, #17107, .T. ) ;
#8151=DIRECTION ( 'NONE',  ( 1.000000000000000000, 1.836970198721030181E-16, 0.000000000000000000 ) ) ;
#8200=ORIENTED_EDGE ( 'NONE', *, *, #10443, .F. ) ;
#8206=FACE_BOUND ( 'NONE', #17081, .T. ) ;
#8219=EDGE_LOOP ( 'NONE', ( #11928, #4385, #8729, #16345, #15842, #734, #11962, #18193 ) ) ;
#8229=FACE_BOUND ( 'NONE', #17260, .T. ) ;
#8284=DIRECTION ( 'NONE',  ( 1.000000000000000000, -1.836970198721030181E-16, -0.000000000000000000 ) ) ;
#8318=DIRECTION ( 'NONE',  ( 1.000000000000000000, 1.836970198721030181E-16, 0.000000000000000000 ) ) ;
#8326=ADVANCED_FACE ( 'NONE', ( #25628 ), #3522, .F. ) ;
#8335=EDGE_CURVE ( 'NONE', #6393, #23049, #15612, .T. ) ;
#8363=FACE_BOUND ( 'NONE', #5748, .T. ) ;
#8412=DIRECTION ( 'NONE',  ( 0.000000000000000000, 1.000000000000000000, 0.000000000000000000 ) ) ;
#8430=VERTEX_POINT ( 'NONE', #8571 ) ;
#8432=ORIENTED_EDGE ( 'NONE', *, *, #23306, .F. ) ;
#8469=FACE_OUTER_BOUND ( 'NONE', #20313, .T. ) ;
#8473=CIRCLE ( 'NONE', #20400, 69.99999999999998579 ) ;
#8497=ORIENTED_EDGE ( 'NONE', *, *, #25450, .T. ) ;
#8499=CYLINDRICAL_SURFACE ( 'NONE', #24503, 30.00000000000000711 ) ;
#8500=ORIENTED_EDGE ( 'NONE', *, *, #21918, .T. ) ;
#8520=DIRECTION ( 'NONE',  ( -1.000000000000000000, 1.836970198721030181E-16, 0.000000000000000000 ) ) ;
#8531=ORIENTED_EDGE ( 'NONE', *, *, #9075, .F. ) ;
#8536=ORIENTED_EDGE ( 'NONE', *, *, #24755, .T. ) ;
#8550=CARTESIAN_POINT ( 'NONE',  ( 200.0000000000000000, -52.49999999999992895, -52.49999999999999289 ) ) ;
#8562=AXIS2_PLACEMENT_3D ( 'NONE', #171, #16265, #24394 ) ;
#8571=CARTESIAN_POINT ( 'NONE',  ( -200.0000000000000000, 61.50000000000009948, -66.50000000000005684 ) ) ;
#8575=ADVANCED_FACE ( 'NONE', ( #23091 ), #17084, .T. ) ;
#8588=ADVANCED_FACE ( 'NONE', ( #13345 ), #25085, .F. ) ;
#8610=CARTESIAN_POINT ( 'NONE',  ( -200.0000000000000000, -52.49999999999970868, 82.49999999999998579 ) ) ;
#8637=EDGE_CURVE ( 'NONE', #20847, #7865, #1085, .T. ) ;
#8682=EDGE_CURVE ( 'NONE', #23802, #18072, #13389, .T. ) ;
#8729=ORIENTED_EDGE ( 'NONE', *, *, #23316, .F. ) ;
#8747=AXIS2_PLACEMENT_3D ( 'NONE', #22162, #24555, #14162 ) ;
#8748=VECTOR ( 'NONE', #25709, 1000.000000000000000 ) ;
#8803=VERTEX_POINT ( 'NONE', #5367 ) ;
#8838=CARTESIAN_POINT ( 'NONE',  ( 190.0000000000000000, -74.99999999999988631, 0.000000000000000000 ) ) ;
#8843=DIRECTION ( 'NONE',  ( 0.000000000000000000, -1.000000000000000000, 0.000000000000000000 ) ) ;
#8862=VERTEX_POINT ( 'NONE', #25722 ) ;
#8867=CARTESIAN_POINT ( 'NONE',  ( 190.0000000000000000, 71.50000000000009948, 66.50000000000005684 ) ) ;
#8871=MANIFOLD_SOLID_BREP ( 'Mirror2', #16424 ) ;
#8896=ORIENTED_EDGE ( 'NONE', *, *, #21527, .F. ) ;
#8983=AXIS2_PLACEMENT_3D ( 'NONE', #2178, #18124, #16129 ) ;
#8990=LINE ( 'NONE', #25101, #19768 ) ;
#8999=ORIENTED_EDGE ( 'NONE', *, *, #13074, .T. ) ;
#9028=VERTEX_POINT ( 'NONE', #3145 ) ;
#9064=LINE ( 'NONE', #17671, #5774 ) ;
#9075=EDGE_CURVE ( 'NONE', #7180, #11718, #18987, .T. ) ;
#9144=EDGE_CURVE ( 'NONE', #60, #19515, #22358, .T. ) ;
#9148=CARTESIAN_POINT ( 'NONE',  ( 190.0000000000000000, -71.50000000000002842, 66.50000000000005684 ) ) ;
#9152=ADVANCED_FACE ( 'NONE', ( #10527 ), #2550, .F. ) ;
#9186=ORIENTED_EDGE ( 'NONE', *, *, #6541, .F. ) ;
#9187=ORIENTED_EDGE ( 'NONE', *, *, #22256, .T. ) ;
#9188=VECTOR ( 'NONE', #16664, 1000.000000000000000 ) ;
#9191=ORIENTED_EDGE ( 'NONE', *, *, #5719, .F. ) ;
#9195=AXIS2_PLACEMENT_3D ( 'NONE', #1577, #11534, #9816 ) ;
#9197=CARTESIAN_POINT ( 'NONE',  ( -190.0000000000000000, -52.49999999999991473, 52.49999999999999289 ) ) ;
#9273=FACE_BOUND ( 'NONE', #4827, .T. ) ;
#9274=DIRECTION ( 'NONE',  ( 0.000000000000000000, -1.000000000000000000, 0.000000000000000000 ) ) ;
#9299=ADVANCED_FACE ( 'NONE', ( #6058 ), #18282, .F. ) ;
#9328=DIRECTION ( 'NONE',  ( 1.000000000000000000, 1.836970198721030181E-16, 0.000000000000000000 ) ) ;
#9336=FACE_OUTER_BOUND ( 'NONE', #18904, .T. ) ;
#9345=LINE ( 'NONE', #7215, #1701 ) ;
#9381=CIRCLE ( 'NONE', #1318, 5.000000000000004441 ) ;
#9382=CIRCLE ( 'NONE', #24276, 29.99999999999999645 ) ;
#9406=VECTOR ( 'NONE', #4971, 1000.000000000000000 ) ;
#9436=ORIENTED_EDGE ( 'NONE', *, *, #8637, .T. ) ;
#9469=EDGE_CURVE ( 'NONE', #4824, #6965, #5758, .T. ) ;
#9474=EDGE_CURVE ( 'NONE', #15543, #18337, #18823, .T. ) ;
#9499=PLANE ( 'NONE',  #14701 ) ;
#9505=CARTESIAN_POINT ( 'NONE',  ( 190.0000000000000000, 66.50000000000009948, -66.50000000000005684 ) ) ;
#9532=LINE ( 'NONE', #9670, #9643 ) ;
#9543=DIRECTION ( 'NONE',  ( 0.000000000000000000, -1.000000000000000000, 0.000000000000000000 ) ) ;
#9573=DIRECTION ( 'NONE',  ( 0.000000000000000000, -1.000000000000000000, 0.000000000000000000 ) ) ;
#9576=DIRECTION ( 'NONE',  ( 1.000000000000000000, -1.836970198721030181E-16, -0.000000000000000000 ) ) ;
#9579=CARTESIAN_POINT ( 'NONE',  ( -190.0000000000000000, -61.50000000000001421, -66.50000000000005684 ) ) ;
#9596=ORIENTED_EDGE ( 'NONE', *, *, #1640, .T. ) ;
#9598=CARTESIAN_POINT ( 'NONE',  ( -190.0000000000000000, -66.50000000000001421, -66.50000000000005684 ) ) ;
#9643=VECTOR ( 'NONE', #24037, 1000.000000000000000 ) ;
#9669=ORIENTED_EDGE ( 'NONE', *, *, #23316, .T. ) ;
#9670=CARTESIAN_POINT ( 'NONE',  ( -190.0000000000000000, 71.50000000000009948, 66.50000000000005684 ) ) ;
#9688=ORIENTED_EDGE ( 'NONE', *, *, #20024, .T. ) ;
#9690=CARTESIAN_POINT ( 'NONE',  ( -200.0000000000000000, 66.50000000000009948, -66.50000000000005684 ) ) ;
#9699=CARTESIAN_POINT ( 'NONE',  ( 190.0000000000000284, -82.49999999999990052, 52.49999999999977973 ) ) ;
#9730=ORIENTED_EDGE ( 'NONE', *, *, #16772, .F. ) ;
#9750=VECTOR ( 'NONE', #11362, 1000.000000000000000 ) ;
#9769=ORIENTED_EDGE ( 'NONE', *, *, #19467, .T. ) ;
#9799=CYLINDRICAL_SURFACE ( 'NONE', #4863, 5.000000000000004441 ) ;
#9806=ADVANCED_FACE ( 'NONE', ( #9880 ), #21725, .F. ) ;
#9816=DIRECTION ( 'NONE',  ( 0.000000000000000000, -1.000000000000000000, 0.000000000000000000 ) ) ;
#9825=VERTEX_POINT ( 'NONE', #3367 ) ;
#9826=DIRECTION ( 'NONE',  ( 0.000000000000000000, -1.000000000000000000, 0.000000000000000000 ) ) ;
#9835=DIRECTION ( 'NONE',  ( 1.836970198721030181E-16, -1.000000000000000000, 1.321694076934715579E-16 ) ) ;
#9838=CIRCLE ( 'NONE', #14939, 5.000000000000004441 ) ;
#9880=FACE_OUTER_BOUND ( 'NONE', #3964, .T. ) ;
#9884=DIRECTION ( 'NONE',  ( 0.000000000000000000, 1.000000000000000000, 0.000000000000000000 ) ) ;
#9889=CARTESIAN_POINT ( 'NONE',  ( -200.0000000000000284, -82.49999999999990052, 52.49999999999977973 ) ) ;
#9932=CARTESIAN_POINT ( 'NONE',  ( 200.0000000000000000, 66.50000000000009948, 66.50000000000005684 ) ) ;
#9956=ORIENTED_EDGE ( 'NONE', *, *, #10708, .F. ) ;
#9995=DIRECTION ( 'NONE',  ( -0.000000000000000000, -1.000000000000000000, -0.000000000000000000 ) ) ;
#10007=EDGE_LOOP ( 'NONE', ( #11646, #19085, #9688, #24519 ) ) ;
#10076=CARTESIAN_POINT ( 'NONE',  ( 190.0000000000000000, 52.49999999999987210, 82.49999999999998579 ) ) ;
#10095=ORIENTED_EDGE ( 'NONE', *, *, #737, .T. ) ;
#10102=ORIENTED_EDGE ( 'NONE', *, *, #3703, .T. ) ;
#10104=CARTESIAN_POINT ( 'NONE',  ( -190.0000000000000000, 66.50000000000009948, 66.50000000000005684 ) ) ;
#10130=LINE ( 'NONE', #18374, #9750 ) ;
#10144=DIRECTION ( 'NONE',  ( 0.000000000000000000, -1.000000000000000000, 0.000000000000000000 ) ) ;
#10222=DIRECTION ( 'NONE',  ( 1.000000000000000000, 0.000000000000000000, -0.000000000000000000 ) ) ;
#10234=ORIENTED_EDGE ( 'NONE', *, *, #8006, .F. ) ;
#10237=DIRECTION ( 'NONE',  ( 0.000000000000000000, -1.000000000000000000, 0.000000000000000000 ) ) ;
#10248=VECTOR ( 'NONE', #25961, 1000.000000000000000 ) ;
#10276=ORIENTED_EDGE ( 'NONE', *, *, #13214, .F. ) ;
#10286=DIRECTION ( 'NONE',  ( 1.000000000000000000, 1.836970198721030181E-16, 0.000000000000000000 ) ) ;
#10291=ADVANCED_FACE ( 'NONE', ( #441, #5092, #23186, #20931, #25316, #11072 ), #10543, .F. ) ;
#10297=EDGE_CURVE ( 'NONE', #12655, #7180, #7222, .T. ) ;
#10309=AXIS2_PLACEMENT_3D ( 'NONE', #9598, #7092, #1370 ) ;
#10334=ORIENTED_EDGE ( 'NONE', *, *, #23713, .T. ) ;
#10341=CARTESIAN_POINT ( 'NONE',  ( 190.0000000000000000, -66.50000000000001421, -66.50000000000005684 ) ) ;
#10363=DIRECTION ( 'NONE',  ( 1.000000000000000000, 1.836970198721030181E-16, 0.000000000000000000 ) ) ;
#10386=CARTESIAN_POINT ( 'NONE',  ( -200.0000000000000000, 69.99999999999995737, 8.572527594031465104E-15 ) ) ;
#10389=EDGE_LOOP ( 'NONE', ( #561, #12002, #19449, #4233 ) ) ;
#10400=ORIENTED_EDGE ( 'NONE', *, *, #3611, .T. ) ;
#10443=EDGE_CURVE ( 'NONE', #24345, #3139, #7319, .T. ) ;
#10444=VECTOR ( 'NONE', #7904, 1000.000000000000000 ) ;
#10455=DIRECTION ( 'NONE',  ( 0.000000000000000000, 1.000000000000000000, 0.000000000000000000 ) ) ;
#10476=DIRECTION ( 'NONE',  ( -1.000000000000000000, -1.836970198721030181E-16, 0.000000000000000000 ) ) ;
#10498=FACE_OUTER_BOUND ( 'NONE', #24249, .T. ) ;
#10499=ORIENTED_EDGE ( 'NONE', *, *, #17902, .F. ) ;
#10527=FACE_OUTER_BOUND ( 'NONE', #3085, .T. ) ;
#10529=ORIENTED_EDGE ( 'NONE', *, *, #12384, .F. ) ;
#10530=ORIENTED_EDGE ( 'NONE', *, *, #8145, .F. ) ;
#10542=LINE ( 'NONE', #25058, #26192 ) ;
#10543=PLANE ( 'NONE',  #16951 ) ;
#10625=EDGE_CURVE ( 'NONE', #15670, #992, #20349, .T. ) ;
#10637=CARTESIAN_POINT ( 'NONE',  ( -190.0000000000000000, -52.49999999999992895, -52.49999999999999289 ) ) ;
#10664=DIRECTION ( 'NONE',  ( 0.000000000000000000, -1.000000000000000000, 0.000000000000000000 ) ) ;
#10694=CARTESIAN_POINT ( 'NONE',  ( -200.0000000000000000, -66.50000000000001421, 66.50000000000005684 ) ) ;
#10700=AXIS2_PLACEMENT_3D ( 'NONE', #22855, #2495, #5026 ) ;
#10703=VERTEX_POINT ( 'NONE', #25926 ) ;
#10708=EDGE_CURVE ( 'NONE', #18643, #9825, #14197, .T. ) ;
#10729=AXIS2_PLACEMENT_3D ( 'NONE', #25229, #484, #21234 ) ;
#10737=ORIENTED_EDGE ( 'NONE', *, *, #1640, .F. ) ;
#10757=DIRECTION ( 'NONE',  ( 1.000000000000000000, -1.836970198721030181E-16, -0.000000000000000000 ) ) ;
#10765=ORIENTED_EDGE ( 'NONE', *, *, #24755, .F. ) ;
#10791=CARTESIAN_POINT ( 'NONE',  ( -190.0000000000000000, 66.50000000000009948, -66.50000000000005684 ) ) ;
#10797=CYLINDRICAL_SURFACE ( 'NONE', #21241, 30.00000000000000355 ) ;
#10885=AXIS2_PLACEMENT_3D ( 'NONE', #25044, #18777, #6662 ) ;
#10897=CIRCLE ( 'NONE', #7470, 5.000000000000004441 ) ;
#10940=AXIS2_PLACEMENT_3D ( 'NONE', #25550, #15166, #23662 ) ;
#10944=CARTESIAN_POINT ( 'NONE',  ( 190.0000000000000000, 61.50000000000009948, 66.50000000000005684 ) ) ;
#10965=ORIENTED_EDGE ( 'NONE', *, *, #16772, .T. ) ;
#10973=ORIENTED_EDGE ( 'NONE', *, *, #25740, .T. ) ;
#10975=VERTEX_POINT ( 'NONE', #17497 ) ;
#11072=FACE_BOUND ( 'NONE', #24172, .T. ) ;
#11096=EDGE_LOOP ( 'NONE', ( #4200, #3546, #7551, #20553 ) ) ;
#11103=CIRCLE ( 'NONE', #17467, 74.99999999999995737 ) ;
#11122=ORIENTED_EDGE ( 'NONE', *, *, #3532, .F. ) ;
#11147=LINE ( 'NONE', #4647, #16184 ) ;
#11148=ORIENTED_EDGE ( 'NONE', *, *, #14182, .F. ) ;
#11152=ORIENTED_EDGE ( 'NONE', *, *, #9144, .F. ) ;
#11167=CYLINDRICAL_SURFACE ( 'NONE', #22144, 5.000000000000004441 ) ;
#11173=VERTEX_POINT ( 'NONE', #18288 ) ;
#11186=FACE_OUTER_BOUND ( 'NONE', #25047, .T. ) ;
#11213=VERTEX_POINT ( 'NONE', #2468 ) ;
#11232=DIRECTION ( 'NONE',  ( 0.000000000000000000, 1.000000000000000000, 0.000000000000000000 ) ) ;
#11265=CARTESIAN_POINT ( 'NONE',  ( -200.0000000000000000, 2.362121657692426575E-30, 0.000000000000000000 ) ) ;
#11266=MECHANICAL_DESIGN_GEOMETRIC_PRESENTATION_REPRESENTATION('',(#24456),#12990);
#11268=CIRCLE ( 'NONE', #12541, 5.000000000000004441 ) ;
#11270=EDGE_LOOP ( 'NONE', ( #24949, #8086 ) ) ;
#11275=ORIENTED_EDGE ( 'NONE', *, *, #6541, .T. ) ;
#11313=AXIS2_PLACEMENT_3D ( 'NONE', #10341, #1971, #1838 ) ;
#11351=CARTESIAN_POINT ( 'NONE',  ( 190.0000000000000000, 52.50000000000007816, 52.49999999999999289 ) ) ;
#11362=DIRECTION ( 'NONE',  ( -0.000000000000000000, -1.000000000000000000, -0.000000000000000000 ) ) ;
#11366=ORIENTED_EDGE ( 'NONE', *, *, #22166, .T. ) ;
#11378=DIRECTION ( 'NONE',  ( 1.836970198721030181E-16, 1.000000000000000000, -1.321694076934715579E-16 ) ) ;
#11419=DIRECTION ( 'NONE',  ( 0.000000000000000000, -0.000000000000000000, 1.000000000000000000 ) ) ;
#11425=ORIENTED_EDGE ( 'NONE', *, *, #19566, .T. ) ;
#11426=DIRECTION ( 'NONE',  ( -0.000000000000000000, -1.321694076934715579E-16, -1.000000000000000000 ) ) ;
#11430=ORIENTED_EDGE ( 'NONE', *, *, #19467, .F. ) ;
#11445=CARTESIAN_POINT ( 'NONE',  ( 200.0000000000000284, -82.49999999999990052, 52.49999999999977973 ) ) ;
#11500=ADVANCED_BREP_SHAPE_REPRESENTATION ( '', ( #8871, #21058 ), #7428 ) ;
#11512=FACE_BOUND ( 'NONE', #15071, .T. ) ;
#11517=ORIENTED_EDGE ( 'NONE', *, *, #7185, .T. ) ;
#11534=DIRECTION ( 'NONE',  ( 1.000000000000000000, 1.836970198721030181E-16, -0.000000000000000000 ) ) ;
#11549=ORIENTED_EDGE ( 'NONE', *, *, #13205, .T. ) ;
#11550=AXIS2_PLACEMENT_3D ( 'NONE', #7338, #1110, #5109 ) ;
#11561=DIRECTION ( 'NONE',  ( 1.000000000000000000, 1.836970198721030181E-16, -0.000000000000000000 ) ) ;
#11567=DIRECTION ( 'NONE',  ( -1.000000000000000000, 1.836970198721030181E-16, 0.000000000000000000 ) ) ;
#11594=EDGE_CURVE ( 'NONE', #6393, #19936, #22057, .T. ) ;
#11611=CYLINDRICAL_SURFACE ( 'NONE', #3616, 29.99999999999999645 ) ;
#11646=ORIENTED_EDGE ( 'NONE', *, *, #12245, .F. ) ;
#11649=DIRECTION ( 'NONE',  ( 1.000000000000000000, 1.836970198721030181E-16, 0.000000000000000000 ) ) ;
#11663=DIRECTION ( 'NONE',  ( 0.000000000000000000, -1.000000000000000000, 0.000000000000000000 ) ) ;
#11681=ORIENTED_EDGE ( 'NONE', *, *, #21128, .F. ) ;
#11693=DIRECTION ( 'NONE',  ( 0.000000000000000000, -1.000000000000000000, 0.000000000000000000 ) ) ;
#11698=CIRCLE ( 'NONE', #21914, 29.99999999999999645 ) ;
#11709=EDGE_CURVE ( 'NONE', #21418, #2760, #23598, .T. ) ;
#11718=VERTEX_POINT ( 'NONE', #7233 ) ;
#11722=CARTESIAN_POINT ( 'NONE',  ( -200.0000000000000000, -52.49999999999970868, 82.49999999999998579 ) ) ;
#11748=DIRECTION ( 'NONE',  ( 1.000000000000000000, -1.836970198721030181E-16, -0.000000000000000000 ) ) ;
#11754=DIRECTION ( 'NONE',  ( 0.000000000000000000, 0.000000000000000000, -1.000000000000000000 ) ) ;
#11765=DIRECTION ( 'NONE',  ( 1.000000000000000000, 1.836970198721030181E-16, -0.000000000000000000 ) ) ;
#11790=CARTESIAN_POINT ( 'NONE',  ( 190.0000000000000284, -82.49999999999990052, 52.49999999999977973 ) ) ;
#11794=ORIENTED_EDGE ( 'NONE', *, *, #21128, .T. ) ;
#11796=DIRECTION ( 'NONE',  ( 0.000000000000000000, 1.000000000000000000, 0.000000000000000000 ) ) ;
#11818=ORIENTED_EDGE ( 'NONE', *, *, #14339, .F. ) ;
#11850=CARTESIAN_POINT ( 'NONE',  ( -200.0000000000000000, 66.50000000000009948, 66.50000000000005684 ) ) ;
#11863=ORIENTED_EDGE ( 'NONE', *, *, #737, .F. ) ;
#11885=CARTESIAN_POINT ( 'NONE',  ( 189.9999999999999716, 82.50000000000008527, 52.49999999999977973 ) ) ;
#11900=EDGE_CURVE ( 'NONE', #19485, #3139, #14400, .T. ) ;
#11928=ORIENTED_EDGE ( 'NONE', *, *, #17606, .F. ) ;
#11962=ORIENTED_EDGE ( 'NONE', *, *, #16617, .F. ) ;
#12002=ORIENTED_EDGE ( 'NONE', *, *, #17510, .T. ) ;
#12045=CARTESIAN_POINT ( 'NONE',  ( -200.0000000000000000, -61.50000000000001421, -66.50000000000005684 ) ) ;
#12069=FACE_BOUND ( 'NONE', #22519, .T. ) ;
#12088=ORIENTED_EDGE ( 'NONE', *, *, #12837, .T. ) ;
#12097=FACE_OUTER_BOUND ( 'NONE', #10389, .T. ) ;
#12114=FACE_OUTER_BOUND ( 'NONE', #7659, .T. ) ;
#12139=PRODUCT_DEFINITION_FORMATION_WITH_SPECIFIED_SOURCE ( 'ANY', '', #24865, .NOT_KNOWN. ) ;
#12145=CIRCLE ( 'NONE', #694, 74.99999999999995737 ) ;
#12148=CYLINDRICAL_SURFACE ( 'NONE', #20273, 5.000000000000004441 ) ;
#12163=ORIENTED_EDGE ( 'NONE', *, *, #17902, .T. ) ;
#12169=SHAPE_REPRESENTATION ( 'Discharge flange', ( #21058 ), #7428 ) ;
#12245=EDGE_CURVE ( 'NONE', #18072, #4824, #23569, .T. ) ;
#12255=ORIENTED_EDGE ( 'NONE', *, *, #631, .F. ) ;
#12260=CARTESIAN_POINT ( 'NONE',  ( -200.0000000000000000, 2.362121657692426575E-30, 0.000000000000000000 ) ) ;
#12277=CARTESIAN_POINT ( 'NONE',  ( 190.0000000000000000, 7.164183775012017527E-14, 0.000000000000000000 ) ) ;
#12347=ORIENTED_EDGE ( 'NONE', *, *, #22794, .F. ) ;
#12362=VECTOR ( 'NONE', #4302, 1000.000000000000000 ) ;
#12363=AXIS2_PLACEMENT_3D ( 'NONE', #24628, #22506, #20501 ) ;
#12382=DIRECTION ( 'NONE',  ( -1.000000000000000000, 1.836970198721030181E-16, 0.000000000000000000 ) ) ;
#12384=EDGE_CURVE ( 'NONE', #17327, #993, #23414, .T. ) ;
#12418=CARTESIAN_POINT ( 'NONE',  ( 200.0000000000000000, -66.50000000000001421, -66.50000000000005684 ) ) ;
#12423=ORIENTED_EDGE ( 'NONE', *, *, #13205, .F. ) ;
#12449=CARTESIAN_POINT ( 'NONE',  ( 190.0000000000000000, 7.164183775012017527E-14, 0.000000000000000000 ) ) ;
#12477=ORIENTED_EDGE ( 'NONE', *, *, #8006, .T. ) ;
#12497=CARTESIAN_POINT ( 'NONE',  ( -199.9999999999999716, 82.50000000000008527, 52.49999999999977973 ) ) ;
#12528=ADVANCED_FACE ( 'NONE', ( #12114 ), #14237, .T. ) ;
#12541=AXIS2_PLACEMENT_3D ( 'NONE', #10694, #8284, #20538 ) ;
#12543=CARTESIAN_POINT ( 'NONE',  ( 190.0000000000000000, -52.49999999999972289, -82.49999999999998579 ) ) ;
#12589=AXIS2_PLACEMENT_3D ( 'NONE', #2362, #10476, #26331 ) ;
#12590=EDGE_LOOP ( 'NONE', ( #11275, #948 ) ) ;
#12627=CIRCLE ( 'NONE', #19367, 30.00000000000000355 ) ;
#12655=VERTEX_POINT ( 'NONE', #18897 ) ;
#12690=EDGE_LOOP ( 'NONE', ( #25181, #3990, #20917, #24205 ) ) ;
#12717=AXIS2_PLACEMENT_3D ( 'NONE', #1604, #3588, #25957 ) ;
#12733=LINE ( 'NONE', #8610, #18754 ) ;
#12753=CARTESIAN_POINT ( 'NONE',  ( 200.0000000000000000, 52.49999999999987210, 82.49999999999998579 ) ) ;
#12756=EDGE_LOOP ( 'NONE', ( #6435, #3326, #2557, #5642, #22848, #8497, #16119, #18500 ) ) ;
#12802=VECTOR ( 'NONE', #12862, 1000.000000000000000 ) ;
#12803=CIRCLE ( 'NONE', #8983, 5.000000000000004441 ) ;
#12813=DIRECTION ( 'NONE',  ( 0.000000000000000000, -1.000000000000000000, 0.000000000000000000 ) ) ;
#12824=ADVANCED_FACE ( 'NONE', ( #21291 ), #11167, .F. ) ;
#12837=EDGE_CURVE ( 'NONE', #15543, #18643, #14058, .T. ) ;
#12858=EDGE_LOOP ( 'NONE', ( #14220, #22124 ) ) ;
#12862=DIRECTION ( 'NONE',  ( 1.000000000000000000, 1.836970198721030181E-16, 0.000000000000000000 ) ) ;
#12990=( GEOMETRIC_REPRESENTATION_CONTEXT ( 3 ) GLOBAL_UNCERTAINTY_ASSIGNED_CONTEXT ( ( #5552 ) ) GLOBAL_UNIT_ASSIGNED_CONTEXT ( ( #5889, #8144, #14398 ) ) REPRESENTATION_CONTEXT ( 'NONE', 'WORKASPACE' ) );
#13004=DIRECTION ( 'NONE',  ( 1.000000000000000000, 1.836970198721030181E-16, 0.000000000000000000 ) ) ;
#13008=CARTESIAN_POINT ( 'NONE',  ( -190.0000000000000284, -82.49999999999990052, 52.49999999999977973 ) ) ;
#13017=DIRECTION ( 'NONE',  ( 0.000000000000000000, -1.000000000000000000, 0.000000000000000000 ) ) ;
#13051=ORIENTED_EDGE ( 'NONE', *, *, #4702, .F. ) ;
#13060=DIRECTION ( 'NONE',  ( 1.000000000000000000, -1.836970198721030181E-16, -0.000000000000000000 ) ) ;
#13074=EDGE_CURVE ( 'NONE', #23831, #11213, #12803, .T. ) ;
#13089=ORIENTED_EDGE ( 'NONE', *, *, #23903, .F. ) ;
#13098=VERTEX_POINT ( 'NONE', #5895 ) ;
#13105=CARTESIAN_POINT ( 'NONE',  ( 200.0000000000000000, -52.49999999999972289, -82.49999999999998579 ) ) ;
#13119=AXIS2_PLACEMENT_3D ( 'NONE', #13317, #3210, #1474 ) ;
#13127=CARTESIAN_POINT ( 'NONE',  ( 190.0000000000000000, -61.50000000000001421, -66.50000000000005684 ) ) ;
#13148=ORIENTED_EDGE ( 'NONE', *, *, #21918, .F. ) ;
#13154=CARTESIAN_POINT ( 'NONE',  ( -190.0000000000000000, -66.50000000000001421, 66.50000000000005684 ) ) ;
#13177=CARTESIAN_POINT ( 'NONE',  ( 199.9999999999999716, 82.50000000000008527, -52.49999999999977973 ) ) ;
#13200=LINE ( 'NONE', #21060, #19378 ) ;
#13205=EDGE_CURVE ( 'NONE', #2384, #3446, #9381, .T. ) ;
#13206=DIRECTION ( 'NONE',  ( 0.000000000000000000, 1.000000000000000000, 0.000000000000000000 ) ) ;
#13211=DIRECTION ( 'NONE',  ( 0.000000000000000000, -1.000000000000000000, 0.000000000000000000 ) ) ;
#13214=EDGE_CURVE ( 'NONE', #3139, #19485, #19586, .T. ) ;
#13231=VECTOR ( 'NONE', #8130, 1000.000000000000000 ) ;
#13290=DIRECTION ( 'NONE',  ( 1.000000000000000000, -1.836970198721030181E-16, -0.000000000000000000 ) ) ;
#13301=EDGE_CURVE ( 'NONE', #9028, #14209, #6021, .T. ) ;
#13312=CARTESIAN_POINT ( 'NONE',  ( -190.0000000000000000, 66.50000000000009948, -66.50000000000005684 ) ) ;
#13317=CARTESIAN_POINT ( 'NONE',  ( 190.0000000000000000, -66.50000000000001421, -66.50000000000005684 ) ) ;
#13345=FACE_OUTER_BOUND ( 'NONE', #25687, .T. ) ;
#13368=EDGE_CURVE ( 'NONE', #433, #17301, #14073, .T. ) ;
#13381=LINE ( 'NONE', #17622, #20620 ) ;
#13387=FACE_BOUND ( 'NONE', #23050, .T. ) ;
#13389=CIRCLE ( 'NONE', #15504, 30.00000000000000355 ) ;
#13444=EDGE_CURVE ( 'NONE', #10703, #14209, #6682, .T. ) ;
#13460=ORIENTED_EDGE ( 'NONE', *, *, #7406, .F. ) ;
#13556=ORIENTED_EDGE ( 'NONE', *, *, #13444, .T. ) ;
#13594=CIRCLE ( 'NONE', #17415, 5.000000000000004441 ) ;
#13646=CIRCLE ( 'NONE', #15764, 5.000000000000004441 ) ;
#13674=CARTESIAN_POINT ( 'NONE',  ( 190.0000000000000000, -52.49999999999970868, 82.49999999999998579 ) ) ;
#13685=CARTESIAN_POINT ( 'NONE',  ( -190.0000000000000000, -52.49999999999972289, -82.49999999999998579 ) ) ;
#13694=CARTESIAN_POINT ( 'NONE',  ( 200.0000000000000000, -66.50000000000001421, 66.50000000000005684 ) ) ;
#13730=DIRECTION ( 'NONE',  ( 0.000000000000000000, -1.000000000000000000, 0.000000000000000000 ) ) ;
#13733=DIRECTION ( 'NONE',  ( 0.000000000000000000, -1.000000000000000000, 0.000000000000000000 ) ) ;
#13748=ORIENTED_EDGE ( 'NONE', *, *, #19163, .T. ) ;
#13757=LINE ( 'NONE', #21753, #2379 ) ;
#13769=DIRECTION ( 'NONE',  ( 0.000000000000000000, 1.000000000000000000, 0.000000000000000000 ) ) ;
#13783=DIRECTION ( 'NONE',  ( 1.000000000000000000, -1.836970198721030181E-16, -0.000000000000000000 ) ) ;
#13819=CARTESIAN_POINT ( 'NONE',  ( 190.0000000000000000, -52.49999999999991473, 52.49999999999999289 ) ) ;
#13823=CARTESIAN_POINT ( 'NONE',  ( 200.0000000000000000, 82.50000000000008527, 52.49999999999979394 ) ) ;
#13851=EDGE_CURVE ( 'NONE', #8803, #19588, #12733, .T. ) ;
#13859=ADVANCED_FACE ( 'NONE', ( #8469 ), #6741, .F. ) ;
#13882=DIRECTION ( 'NONE',  ( -1.000000000000000000, 0.000000000000000000, -0.000000000000000000 ) ) ;
#13953=ORIENTED_EDGE ( 'NONE', *, *, #4520, .T. ) ;
#13976=DIRECTION ( 'NONE',  ( 1.000000000000000000, -1.836970198721030181E-16, -0.000000000000000000 ) ) ;
#13978=VECTOR ( 'NONE', #19439, 1000.000000000000000 ) ;
#14018=AXIS2_PLACEMENT_3D ( 'NONE', #18655, #22795, #4966 ) ;
#14050=ORIENTED_EDGE ( 'NONE', *, *, #7185, .F. ) ;
#14058=CIRCLE ( 'NONE', #22586, 74.99999999999995737 ) ;
#14073=CIRCLE ( 'NONE', #25992, 30.00000000000000355 ) ;
#14091=CIRCLE ( 'NONE', #24309, 30.00000000000000355 ) ;
#14161=FACE_OUTER_BOUND ( 'NONE', #11096, .T. ) ;
#14162=DIRECTION ( 'NONE',  ( 0.000000000000000000, 1.000000000000000000, 0.000000000000000000 ) ) ;
#14180=VERTEX_POINT ( 'NONE', #4468 ) ;
#14182=EDGE_CURVE ( 'NONE', #6305, #218, #22828, .T. ) ;
#14187=ORIENTED_EDGE ( 'NONE', *, *, #10625, .T. ) ;
#14196=FACE_BOUND ( 'NONE', #22876, .T. ) ;
#14197=LINE ( 'NONE', #17917, #5050 ) ;
#14209=VERTEX_POINT ( 'NONE', #13105 ) ;
#14211=DIRECTION ( 'NONE',  ( 1.000000000000000000, -1.836970198721030181E-16, -0.000000000000000000 ) ) ;
#14220=ORIENTED_EDGE ( 'NONE', *, *, #8637, .F. ) ;
#14237=CYLINDRICAL_SURFACE ( 'NONE', #12363, 29.99999999999999289 ) ;
#14250=( NAMED_UNIT ( * ) PLANE_ANGLE_UNIT ( ) SI_UNIT ( $, .RADIAN. ) );
#14269=VECTOR ( 'NONE', #21023, 1000.000000000000000 ) ;
#14331=ADVANCED_FACE ( 'NONE', ( #17724 ), #23595, .F. ) ;
#14339=EDGE_CURVE ( 'NONE', #19588, #21418, #25374, .T. ) ;
#14346=ADVANCED_FACE ( 'NONE', ( #23719 ), #5500, .T. ) ;
#14353=ORIENTED_EDGE ( 'NONE', *, *, #2792, .T. ) ;
#14358=CARTESIAN_POINT ( 'NONE',  ( -190.0000000000000284, -82.49999999999990052, 52.49999999999977973 ) ) ;
#14381=ORIENTED_EDGE ( 'NONE', *, *, #16617, .T. ) ;
#14398=( NAMED_UNIT ( * ) SI_UNIT ( $, .STERADIAN. ) SOLID_ANGLE_UNIT ( ) );
#14400=CIRCLE ( 'NONE', #19917, 5.000000000000004441 ) ;
#14456=LINE ( 'NONE', #20721, #20874 ) ;
#14484=ADVANCED_FACE ( 'NONE', ( #3772 ), #12148, .F. ) ;
#14543=CARTESIAN_POINT ( 'NONE',  ( -190.0000000000000000, 52.50000000000007816, -52.49999999999999289 ) ) ;
#14560=CARTESIAN_POINT ( 'NONE',  ( -200.0000000000000000, -71.50000000000002842, 66.50000000000005684 ) ) ;
#14585=DIRECTION ( 'NONE',  ( 0.000000000000000000, -1.000000000000000000, 0.000000000000000000 ) ) ;
#14605=ORIENTED_EDGE ( 'NONE', *, *, #5075, .F. ) ;
#14622=LINE ( 'NONE', #20761, #14689 ) ;
#14689=VECTOR ( 'NONE', #19025, 1000.000000000000000 ) ;
#14701=AXIS2_PLACEMENT_3D ( 'NONE', #15362, #11754, #13882 ) ;
#14747=CARTESIAN_POINT ( 'NONE',  ( -190.0000000000000000, 52.49999999999987210, 82.49999999999998579 ) ) ;
#14780=ORIENTED_EDGE ( 'NONE', *, *, #21855, .F. ) ;
#14781=CARTESIAN_POINT ( 'NONE',  ( -190.0000000000000000, -66.50000000000001421, -66.50000000000005684 ) ) ;
#14793=DIRECTION ( 'NONE',  ( 1.000000000000000000, 1.836970198721030181E-16, 0.000000000000000000 ) ) ;
#14845=ORIENTED_EDGE ( 'NONE', *, *, #23306, .T. ) ;
#14846=LINE ( 'NONE', #8867, #12802 ) ;
#14853=EDGE_CURVE ( 'NONE', #555, #19588, #14898, .T. ) ;
#14855=DIRECTION ( 'NONE',  ( 0.000000000000000000, 1.000000000000000000, 0.000000000000000000 ) ) ;
#14898=LINE ( 'NONE', #4288, #4140 ) ;
#14939=AXIS2_PLACEMENT_3D ( 'NONE', #4657, #531, #4529 ) ;
#14951=ORIENTED_EDGE ( 'NONE', *, *, #6156, .F. ) ;
#14953=ORIENTED_EDGE ( 'NONE', *, *, #25263, .T. ) ;
#14956=AXIS2_PLACEMENT_3D ( 'NONE', #21936, #11419, #25940 ) ;
#14988=FACE_OUTER_BOUND ( 'NONE', #20214, .T. ) ;
#15011=EDGE_CURVE ( 'NONE', #19936, #17205, #2277, .T. ) ;
#15023=DIRECTION ( 'NONE',  ( 0.000000000000000000, -1.000000000000000000, 0.000000000000000000 ) ) ;
#15061=DIRECTION ( 'NONE',  ( 0.000000000000000000, 1.000000000000000000, 0.000000000000000000 ) ) ;
#15069=PLANE ( 'NONE',  #25318 ) ;
#15071=EDGE_LOOP ( 'NONE', ( #2727, #12088 ) ) ;
#15088=DIRECTION ( 'NONE',  ( 0.000000000000000000, -1.000000000000000000, 0.000000000000000000 ) ) ;
#15095=ADVANCED_FACE ( 'NONE', ( #18633 ), #2684, .F. ) ;
#15108=DIRECTION ( 'NONE',  ( 1.000000000000000000, 1.836970198721030181E-16, 0.000000000000000000 ) ) ;
#15113=AXIS2_PLACEMENT_3D ( 'NONE', #17627, #17504, #13769 ) ;
#15134=CARTESIAN_POINT ( 'NONE',  ( -190.0000000000000000, 1.836970198721033928E-15, 0.000000000000000000 ) ) ;
#15158=ADVANCED_FACE ( 'NONE', ( #25673 ), #5193, .F. ) ;
#15166=DIRECTION ( 'NONE',  ( 1.000000000000000000, 1.836970198721030181E-16, 0.000000000000000000 ) ) ;
#15240=CARTESIAN_POINT ( 'NONE',  ( 200.0000000000000000, 66.50000000000009948, -66.50000000000005684 ) ) ;
#15250=EDGE_CURVE ( 'NONE', #15670, #11173, #23788, .T. ) ;
#15269=DIRECTION ( 'NONE',  ( 0.000000000000000000, -1.000000000000000000, 0.000000000000000000 ) ) ;
#15311=AXIS2_PLACEMENT_3D ( 'NONE', #9197, #5459, #9573 ) ;
#15332=ORIENTED_EDGE ( 'NONE', *, *, #5390, .F. ) ;
#15344=PRODUCT_DEFINITION_CONTEXT ( 'detailed design', #2056, 'design' ) ;
#15348=CIRCLE ( 'NONE', #6842, 5.000000000000004441 ) ;
#15362=CARTESIAN_POINT ( 'NONE',  ( -190.0000000000000000, -52.49999999999970868, 82.49999999999998579 ) ) ;
#15365=ORIENTED_EDGE ( 'NONE', *, *, #3611, .F. ) ;
#15368=CARTESIAN_POINT ( 'NONE',  ( 190.0000000000000000, 52.49999999999987210, 82.49999999999998579 ) ) ;
#15381=CIRCLE ( 'NONE', #3934, 5.000000000000004441 ) ;
#15394=ORIENTED_EDGE ( 'NONE', *, *, #12837, .F. ) ;
#15451=CARTESIAN_POINT ( 'NONE',  ( -200.0000000000000000, -71.50000000000002842, -66.50000000000005684 ) ) ;
#15504=AXIS2_PLACEMENT_3D ( 'NONE', #24119, #15589, #7604 ) ;
#15535=ORIENTED_EDGE ( 'NONE', *, *, #631, .T. ) ;
#15543=VERTEX_POINT ( 'NONE', #17143 ) ;
#15548=ORIENTED_EDGE ( 'NONE', *, *, #8335, .T. ) ;
#15551=DIRECTION ( 'NONE',  ( 1.000000000000000000, -1.836970198721030181E-16, -0.000000000000000000 ) ) ;
#15589=DIRECTION ( 'NONE',  ( 1.000000000000000000, 1.836970198721030181E-16, -0.000000000000000000 ) ) ;
#15612=LINE ( 'NONE', #21618, #18052 ) ;
#15630=CARTESIAN_POINT ( 'NONE',  ( 190.0000000000000000, -52.49999999999992895, -52.49999999999999289 ) ) ;
#15650=UNCERTAINTY_MEASURE_WITH_UNIT (LENGTH_MEASURE( 1.000000000000000082E-05 ), #4028, 'distance_accuracy_value', 'NONE');
#15670=VERTEX_POINT ( 'NONE', #13127 ) ;
#15673=AXIS2_PLACEMENT_3D ( 'NONE', #13674, #17792, #10222 ) ;
#15681=DIRECTION ( 'NONE',  ( 0.000000000000000000, -1.000000000000000000, 0.000000000000000000 ) ) ;
#15684=LINE ( 'NONE', #3467, #10248 ) ;
#15693=VECTOR ( 'NONE', #23044, 1000.000000000000000 ) ;
#15738=ORIENTED_EDGE ( 'NONE', *, *, #12245, .T. ) ;
#15744=AXIS2_PLACEMENT_3D ( 'NONE', #17566, #5600, #5221 ) ;
#15764=AXIS2_PLACEMENT_3D ( 'NONE', #7439, #15551, #23678 ) ;
#15771=EDGE_LOOP ( 'NONE', ( #9596, #22398 ) ) ;
#15780=DIRECTION ( 'NONE',  ( 1.000000000000000000, 1.836970198721030181E-16, -0.000000000000000000 ) ) ;
#15781=EDGE_CURVE ( 'NONE', #23831, #23552, #13757, .T. ) ;
#15794=EDGE_CURVE ( 'NONE', #17327, #60, #18015, .T. ) ;
#15842=ORIENTED_EDGE ( 'NONE', *, *, #13368, .F. ) ;
#15875=DIRECTION ( 'NONE',  ( 0.000000000000000000, -1.000000000000000000, 0.000000000000000000 ) ) ;
#15932=ORIENTED_EDGE ( 'NONE', *, *, #2672, .F. ) ;
#15941=AXIS2_PLACEMENT_3D ( 'NONE', #4071, #20293, #4731 ) ;
#15942=CIRCLE ( 'NONE', #4502, 5.000000000000004441 ) ;
#15958=CIRCLE ( 'NONE', #6626, 5.000000000000004441 ) ;
#15977=DIRECTION ( 'NONE',  ( 1.000000000000000000, 0.000000000000000000, 0.000000000000000000 ) ) ;
#15990=AXIS2_PLACEMENT_3D ( 'NONE', #6255, #6379, #269 ) ;
#16044=CARTESIAN_POINT ( 'NONE',  ( 190.0000000000000000, 52.49999999999987210, -82.49999999999998579 ) ) ;
#16106=CIRCLE ( 'NONE', #1303, 5.000000000000004441 ) ;
#16114=ORIENTED_EDGE ( 'NONE', *, *, #17515, .F. ) ;
#16119=ORIENTED_EDGE ( 'NONE', *, *, #23402, .T. ) ;
#16129=DIRECTION ( 'NONE',  ( 0.000000000000000000, 1.000000000000000000, 0.000000000000000000 ) ) ;
#16163=CIRCLE ( 'NONE', #21273, 5.000000000000004441 ) ;
#16176=EDGE_LOOP ( 'NONE', ( #2321, #7307 ) ) ;
#16184=VECTOR ( 'NONE', #17001, 1000.000000000000000 ) ;
#16217=VERTEX_POINT ( 'NONE', #14560 ) ;
#16251=ORIENTED_EDGE ( 'NONE', *, *, #2256, .T. ) ;
#16265=DIRECTION ( 'NONE',  ( 1.000000000000000000, -1.836970198721030181E-16, -0.000000000000000000 ) ) ;
#16345=ORIENTED_EDGE ( 'NONE', *, *, #24526, .F. ) ;
#16347=CARTESIAN_POINT ( 'NONE',  ( -190.0000000000000000, 52.49999999999987210, -82.49999999999998579 ) ) ;
#16368=CIRCLE ( 'NONE', #23188, 69.99999999999998579 ) ;
#16370=DIRECTION ( 'NONE',  ( -1.000000000000000000, 1.836970198721030181E-16, 0.000000000000000000 ) ) ;
#16378=SHAPE_REPRESENTATION_RELATIONSHIP ( 'NONE' , 'NONE' ,  #12169, #11500 ) ;
#16424=CLOSED_SHELL ( 'NONE', ( #9152, #19460, #21274, #13859, #15158, #17292, #8326, #7194, #9806, #8575, #5720, #10291, #23166, #17427, #1772, #193, #3968, #23755, #14346, #4223, #304, #26165, #20798, #17741, #23538, #9299, #12824, #300, #1053, #18250, #24702, #14331, #21016, #5912, #12528, #2006, #21811, #15095, #8588, #14484 ) ) ;
#16428=AXIS2_PLACEMENT_3D ( 'NONE', #21600, #19221, #3373 ) ;
#16450=VECTOR ( 'NONE', #18192, 1000.000000000000000 ) ;
#16508=CARTESIAN_POINT ( 'NONE',  ( 190.0000000000000000, -66.50000000000001421, 66.50000000000005684 ) ) ;
#16516=ORIENTED_EDGE ( 'NONE', *, *, #13851, .T. ) ;
#16525=FACE_OUTER_BOUND ( 'NONE', #25994, .T. ) ;
#16552=VERTEX_POINT ( 'NONE', #17783 ) ;
#16588=DIRECTION ( 'NONE',  ( 0.000000000000000000, -1.000000000000000000, -0.000000000000000000 ) ) ;
#16612=DIRECTION ( 'NONE',  ( 0.000000000000000000, 1.000000000000000000, 0.000000000000000000 ) ) ;
#16613=ORIENTED_EDGE ( 'NONE', *, *, #9469, .T. ) ;
#16617=EDGE_CURVE ( 'NONE', #20651, #24679, #12627, .T. ) ;
#16638=DIRECTION ( 'NONE',  ( 0.000000000000000000, -1.000000000000000000, 0.000000000000000000 ) ) ;
#16664=DIRECTION ( 'NONE',  ( 1.000000000000000000, 1.836970198721030181E-16, 0.000000000000000000 ) ) ;
#16720=CARTESIAN_POINT ( 'NONE',  ( 190.0000000000000000, 66.50000000000009948, 66.50000000000005684 ) ) ;
#16772=EDGE_CURVE ( 'NONE', #12655, #14180, #10542, .T. ) ;
#16781=EDGE_LOOP ( 'NONE', ( #5871, #17713, #15548, #26081 ) ) ;
#16791=CARTESIAN_POINT ( 'NONE',  ( -200.0000000000000000, 75.00000000000000000, 0.000000000000000000 ) ) ;
#16865=CARTESIAN_POINT ( 'NONE',  ( -199.9999999999999716, 82.50000000000008527, -52.49999999999977973 ) ) ;
#16871=CARTESIAN_POINT ( 'NONE',  ( 200.0000000000000000, 52.49999999999987210, -82.49999999999998579 ) ) ;
#16894=CARTESIAN_POINT ( 'NONE',  ( 190.0000000000000000, 82.50000000000008527, 52.49999999999979394 ) ) ;
#16911=ORIENTED_EDGE ( 'NONE', *, *, #2240, .F. ) ;
#16937=DIRECTION ( 'NONE',  ( 0.000000000000000000, 0.000000000000000000, -1.000000000000000000 ) ) ;
#16947=EDGE_LOOP ( 'NONE', ( #1623, #10095, #13748, #17411 ) ) ;
#16951=AXIS2_PLACEMENT_3D ( 'NONE', #16791, #14793, #971 ) ;
#17001=DIRECTION ( 'NONE',  ( 0.000000000000000000, -1.321694076934715579E-16, -1.000000000000000000 ) ) ;
#17080=EDGE_LOOP ( 'NONE', ( #2655, #13051, #16911, #23111 ) ) ;
#17081=EDGE_LOOP ( 'NONE', ( #21589, #25939 ) ) ;
#17084=CYLINDRICAL_SURFACE ( 'NONE', #24883, 74.99999999999995737 ) ;
#17086=DIRECTION ( 'NONE',  ( -1.000000000000000000, -1.836970198721030181E-16, -0.000000000000000000 ) ) ;
#17107=LINE ( 'NONE', #19238, #3886 ) ;
#17143=CARTESIAN_POINT ( 'NONE',  ( 190.0000000000000000, 75.00000000000004263, 9.184850993605150311E-15 ) ) ;
#17161=ORIENTED_EDGE ( 'NONE', *, *, #15781, .F. ) ;
#17188=DIRECTION ( 'NONE',  ( 0.000000000000000000, -1.321694076934715579E-16, -1.000000000000000000 ) ) ;
#17205=VERTEX_POINT ( 'NONE', #25789 ) ;
#17231=AXIS2_PLACEMENT_3D ( 'NONE', #7541, #21283, #9543 ) ;
#17260=EDGE_LOOP ( 'NONE', ( #14951, #12347 ) ) ;
#17292=ADVANCED_FACE ( 'NONE', ( #24181 ), #3972, .F. ) ;
#17300=ORIENTED_EDGE ( 'NONE', *, *, #4702, .T. ) ;
#17301=VERTEX_POINT ( 'NONE', #10076 ) ;
#17317=CARTESIAN_POINT ( 'NONE',  ( -200.0000000000000000, -52.49999999999972289, -82.49999999999998579 ) ) ;
#17321=DIRECTION ( 'NONE',  ( 1.000000000000000000, 1.836970198721030181E-16, 0.000000000000000000 ) ) ;
#17327=VERTEX_POINT ( 'NONE', #7937 ) ;
#17330=DIRECTION ( 'NONE',  ( 0.000000000000000000, -1.000000000000000000, -0.000000000000000000 ) ) ;
#17359=AXIS2_PLACEMENT_3D ( 'NONE', #7477, #19722, #13730 ) ;
#17375=DIRECTION ( 'NONE',  ( -1.000000000000000000, 1.836970198721030181E-16, 0.000000000000000000 ) ) ;
#17411=ORIENTED_EDGE ( 'NONE', *, *, #15250, .F. ) ;
#17415=AXIS2_PLACEMENT_3D ( 'NONE', #12418, #324, #18269 ) ;
#17427=ADVANCED_FACE ( 'NONE', ( #14196, #12069, #8206, #18450, #20587, #24325 ), #6089, .F. ) ;
#17467=AXIS2_PLACEMENT_3D ( 'NONE', #12449, #5574, #20077 ) ;
#17485=VECTOR ( 'NONE', #18477, 1000.000000000000000 ) ;
#17486=CARTESIAN_POINT ( 'NONE',  ( -190.0000000000000000, 71.50000000000009948, -66.50000000000005684 ) ) ;
#17488=DIRECTION ( 'NONE',  ( -1.000000000000000000, 1.836970198721030181E-16, 0.000000000000000000 ) ) ;
#17493=LINE ( 'NONE', #24258, #21941 ) ;
#17497=CARTESIAN_POINT ( 'NONE',  ( -200.0000000000000000, 71.50000000000009948, 66.50000000000005684 ) ) ;
#17504=DIRECTION ( 'NONE',  ( 1.000000000000000000, 1.836970198721030181E-16, 0.000000000000000000 ) ) ;
#17510=EDGE_CURVE ( 'NONE', #11213, #23831, #10897, .T. ) ;
#17515=EDGE_CURVE ( 'NONE', #13098, #19453, #2636, .T. ) ;
#17566=CARTESIAN_POINT ( 'NONE',  ( 190.0000000000000000, 66.50000000000009948, -66.50000000000005684 ) ) ;
#17577=ORIENTED_EDGE ( 'NONE', *, *, #21527, .T. ) ;
#17583=ORIENTED_EDGE ( 'NONE', *, *, #7406, .T. ) ;
#17606=EDGE_CURVE ( 'NONE', #4564, #10703, #24490, .T. ) ;
#17622=CARTESIAN_POINT ( 'NONE',  ( -190.0000000000000000, -61.50000000000001421, 66.50000000000005684 ) ) ;
#17627=CARTESIAN_POINT ( 'NONE',  ( 190.0000000000000000, -52.49999999999991473, 52.49999999999999289 ) ) ;
#17630=AXIS2_PLACEMENT_3D ( 'NONE', #9505, #24142, #25754 ) ;
#17636=FACE_OUTER_BOUND ( 'NONE', #24901, .T. ) ;
#17670=AXIS2_PLACEMENT_3D ( 'NONE', #9699, #9835, #21946 ) ;
#17671=CARTESIAN_POINT ( 'NONE',  ( -190.0000000000000284, -82.49999999999990052, 52.49999999999977973 ) ) ;
#17712=VECTOR ( 'NONE', #6631, 1000.000000000000000 ) ;
#17713=ORIENTED_EDGE ( 'NONE', *, *, #11594, .F. ) ;
#17724=FACE_OUTER_BOUND ( 'NONE', #20650, .T. ) ;
#17741=ADVANCED_FACE ( 'NONE', ( #14988 ), #6742, .F. ) ;
#17770=DIRECTION ( 'NONE',  ( 1.000000000000000000, 1.836970198721030181E-16, 0.000000000000000000 ) ) ;
#17773=EDGE_LOOP ( 'NONE', ( #25333, #3079, #11425, #25168 ) ) ;
#17783=CARTESIAN_POINT ( 'NONE',  ( -190.0000000000000000, 82.50000000000008527, 52.49999999999979394 ) ) ;
#17792=DIRECTION ( 'NONE',  ( 0.000000000000000000, 0.000000000000000000, 1.000000000000000000 ) ) ;
#17795=DIRECTION ( 'NONE',  ( 1.000000000000000000, 1.836970198721030181E-16, -0.000000000000000000 ) ) ;
#17796=DIRECTION ( 'NONE',  ( 0.000000000000000000, -1.000000000000000000, 0.000000000000000000 ) ) ;
#17809=CARTESIAN_POINT ( 'NONE',  ( -200.0000000000000284, -82.49999999999990052, 52.49999999999977973 ) ) ;
#17841=CARTESIAN_POINT ( 'NONE',  ( 200.0000000000000000, 69.99999999999998579, 8.572527594031466682E-15 ) ) ;
#17902=EDGE_CURVE ( 'NONE', #993, #17327, #4961, .T. ) ;
#17904=DIRECTION ( 'NONE',  ( 0.000000000000000000, 1.000000000000000000, 0.000000000000000000 ) ) ;
#17915=CIRCLE ( 'NONE', #26022, 29.99999999999999289 ) ;
#17917=CARTESIAN_POINT ( 'NONE',  ( -200.0000000000000000, -74.99999999999995737, 0.000000000000000000 ) ) ;
#17932=PRODUCT_CONTEXT ( 'NONE', #17997, 'mechanical' ) ;
#17933=ORIENTED_EDGE ( 'NONE', *, *, #20627, .F. ) ;
#17956=CARTESIAN_POINT ( 'NONE',  ( -190.0000000000000000, 71.50000000000009948, -66.50000000000005684 ) ) ;
#17958=CARTESIAN_POINT ( 'NONE',  ( -200.0000000000000000, 61.50000000000009948, 66.50000000000005684 ) ) ;
#17970=DIRECTION ( 'NONE',  ( -1.000000000000000000, -1.836970198721030181E-16, -0.000000000000000000 ) ) ;
#17972=VERTEX_POINT ( 'NONE', #16865 ) ;
#17977=EDGE_LOOP ( 'NONE', ( #16516, #6701, #4857, #17583 ) ) ;
#17992=DIRECTION ( 'NONE',  ( -0.000000000000000000, -1.321694076934715579E-16, -1.000000000000000000 ) ) ;
#17997=APPLICATION_CONTEXT ( 'automotive_design' ) ;
#17999=DIRECTION ( 'NONE',  ( -1.836970198721030181E-16, 1.000000000000000000, 0.000000000000000000 ) ) ;
#18015=LINE ( 'NONE', #25760, #10444 ) ;
#18037=CARTESIAN_POINT ( 'NONE',  ( 200.0000000000000284, -82.49999999999990052, 52.49999999999977973 ) ) ;
#18038=DIRECTION ( 'NONE',  ( 0.000000000000000000, 1.000000000000000000, 0.000000000000000000 ) ) ;
#18052=VECTOR ( 'NONE', #7898, 1000.000000000000000 ) ;
#18053=CIRCLE ( 'NONE', #1934, 5.000000000000004441 ) ;
#18072=VERTEX_POINT ( 'NONE', #13177 ) ;
#18074=CARTESIAN_POINT ( 'NONE',  ( 200.0000000000000000, 71.50000000000009948, -66.50000000000005684 ) ) ;
#18095=DIRECTION ( 'NONE',  ( -1.000000000000000000, 1.836970198721030181E-16, 0.000000000000000000 ) ) ;
#18124=DIRECTION ( 'NONE',  ( 1.000000000000000000, -1.836970198721030181E-16, -0.000000000000000000 ) ) ;
#18137=AXIS2_PLACEMENT_3D ( 'NONE', #13154, #25145, #15269 ) ;
#18148=CYLINDRICAL_SURFACE ( 'NONE', #21115, 74.99999999999995737 ) ;
#18191=DIRECTION ( 'NONE',  ( -1.000000000000000000, 1.836970198721030181E-16, 0.000000000000000000 ) ) ;
#18192=DIRECTION ( 'NONE',  ( 1.000000000000000000, 1.836970198721030181E-16, 0.000000000000000000 ) ) ;
#18193=ORIENTED_EDGE ( 'NONE', *, *, #1482, .F. ) ;
#18248=DIRECTION ( 'NONE',  ( -1.000000000000000000, 1.836970198721030181E-16, 0.000000000000000000 ) ) ;
#18249=EDGE_CURVE ( 'NONE', #19453, #19106, #17915, .T. ) ;
#18250=ADVANCED_FACE ( 'NONE', ( #1203 ), #3319, .F. ) ;
#18269=DIRECTION ( 'NONE',  ( 0.000000000000000000, 1.000000000000000000, 0.000000000000000000 ) ) ;
#18282=CYLINDRICAL_SURFACE ( 'NONE', #8747, 5.000000000000004441 ) ;
#18288=CARTESIAN_POINT ( 'NONE',  ( 200.0000000000000000, -61.50000000000001421, -66.50000000000005684 ) ) ;
#18300=ORIENTED_EDGE ( 'NONE', *, *, #23402, .F. ) ;
#18336=ORIENTED_EDGE ( 'NONE', *, *, #14853, .T. ) ;
#18337=VERTEX_POINT ( 'NONE', #21673 ) ;
#18374=CARTESIAN_POINT ( 'NONE',  ( 200.0000000000000000, -52.49999999999970868, 82.49999999999998579 ) ) ;
#18376=DIRECTION ( 'NONE',  ( 0.000000000000000000, 1.000000000000000000, 0.000000000000000000 ) ) ;
#18434=VECTOR ( 'NONE', #11649, 1000.000000000000000 ) ;
#18450=FACE_BOUND ( 'NONE', #6278, .T. ) ;
#18472=LINE ( 'NONE', #14747, #17712 ) ;
#18473=FACE_BOUND ( 'NONE', #12590, .T. ) ;
#18477=DIRECTION ( 'NONE',  ( -1.000000000000000000, 1.836970198721030181E-16, 0.000000000000000000 ) ) ;
#18497=DIRECTION ( 'NONE',  ( -1.000000000000000000, -1.836970198721030181E-16, -0.000000000000000000 ) ) ;
#18500=ORIENTED_EDGE ( 'NONE', *, *, #6380, .T. ) ;
#18502=LINE ( 'NONE', #22515, #15693 ) ;
#18546=ORIENTED_EDGE ( 'NONE', *, *, #9075, .T. ) ;
#18633=FACE_OUTER_BOUND ( 'NONE', #2287, .T. ) ;
#18643=VERTEX_POINT ( 'NONE', #8838 ) ;
#18655=CARTESIAN_POINT ( 'NONE',  ( 190.0000000000000000, -66.50000000000001421, 66.50000000000005684 ) ) ;
#18680=VERTEX_POINT ( 'NONE', #2730 ) ;
#18740=CIRCLE ( 'NONE', #1321, 74.99999999999995737 ) ;
#18754=VECTOR ( 'NONE', #16588, 1000.000000000000000 ) ;
#18777=DIRECTION ( 'NONE',  ( -1.000000000000000000, 1.836970198721030181E-16, 0.000000000000000000 ) ) ;
#18779=ORIENTED_EDGE ( 'NONE', *, *, #11900, .F. ) ;
#18800=DIRECTION ( 'NONE',  ( 1.000000000000000000, 1.836970198721030181E-16, -0.000000000000000000 ) ) ;
#18806=CARTESIAN_POINT ( 'NONE',  ( 200.0000000000000000, 71.50000000000009948, 66.50000000000005684 ) ) ;
#18823=LINE ( 'NONE', #20957, #4501 ) ;
#18897=CARTESIAN_POINT ( 'NONE',  ( 190.0000000000000000, -61.50000000000001421, 66.50000000000005684 ) ) ;
#18904=EDGE_LOOP ( 'NONE', ( #12255, #10529, #24814, #7726 ) ) ;
#18932=CARTESIAN_POINT ( 'NONE',  ( 190.0000000000000000, -52.49999999999972289, -82.49999999999998579 ) ) ;
#18987=LINE ( 'NONE', #3271, #21491 ) ;
#19005=AXIS2_PLACEMENT_3D ( 'NONE', #10791, #8520, #16638 ) ;
#19025=DIRECTION ( 'NONE',  ( 1.000000000000000000, 1.836970198721030181E-16, 0.000000000000000000 ) ) ;
#19060=CARTESIAN_POINT ( 'NONE',  ( 190.0000000000000000, 61.50000000000009948, -66.50000000000005684 ) ) ;
#19084=ORIENTED_EDGE ( 'NONE', *, *, #17606, .T. ) ;
#19085=ORIENTED_EDGE ( 'NONE', *, *, #965, .F. ) ;
#19106=VERTEX_POINT ( 'NONE', #18037 ) ;
#19130=CARTESIAN_POINT ( 'NONE',  ( -200.0000000000000000, 52.50000000000007816, -52.49999999999999289 ) ) ;
#19163=EDGE_CURVE ( 'NONE', #2989, #11173, #15381, .T. ) ;
#19184=CARTESIAN_POINT ( 'NONE',  ( -200.0000000000000000, -69.99999999999998579, 0.000000000000000000 ) ) ;
#19206=ORIENTED_EDGE ( 'NONE', *, *, #10297, .F. ) ;
#19220=EDGE_CURVE ( 'NONE', #19936, #6393, #5604, .T. ) ;
#19221=DIRECTION ( 'NONE',  ( -1.836970198721030181E-16, -1.000000000000000000, 0.000000000000000000 ) ) ;
#19238=CARTESIAN_POINT ( 'NONE',  ( -190.0000000000000284, -82.49999999999991473, -52.49999999999977973 ) ) ;
#19279=LINE ( 'NONE', #16894, #14269 ) ;
#19283=CARTESIAN_POINT ( 'NONE',  ( 190.0000000000000000, -66.50000000000001421, 66.50000000000005684 ) ) ;
#19295=ORIENTED_EDGE ( 'NONE', *, *, #4520, .F. ) ;
#19332=ORIENTED_EDGE ( 'NONE', *, *, #11709, .F. ) ;
#19337=DIRECTION ( 'NONE',  ( -1.000000000000000000, 1.836970198721030181E-16, 0.000000000000000000 ) ) ;
#19367=AXIS2_PLACEMENT_3D ( 'NONE', #23908, #15780, #11663 ) ;
#19378=VECTOR ( 'NONE', #9328, 1000.000000000000000 ) ;
#19439=DIRECTION ( 'NONE',  ( 0.000000000000000000, 1.000000000000000000, 0.000000000000000000 ) ) ;
#19449=ORIENTED_EDGE ( 'NONE', *, *, #15781, .T. ) ;
#19453=VERTEX_POINT ( 'NONE', #23334 ) ;
#19460=ADVANCED_FACE ( 'NONE', ( #25335 ), #23457, .F. ) ;
#19467=EDGE_CURVE ( 'NONE', #22119, #21182, #23067, .T. ) ;
#19468=DIRECTION ( 'NONE',  ( 0.000000000000000000, 1.000000000000000000, 0.000000000000000000 ) ) ;
#19479=CARTESIAN_POINT ( 'NONE',  ( -190.0000000000000000, 52.49999999999987210, 82.49999999999998579 ) ) ;
#19485=VERTEX_POINT ( 'NONE', #15451 ) ;
#19507=CARTESIAN_POINT ( 'NONE',  ( -189.9999999999999716, 82.50000000000008527, 52.49999999999977973 ) ) ;
#19515=VERTEX_POINT ( 'NONE', #25712 ) ;
#19538=ORIENTED_EDGE ( 'NONE', *, *, #23713, .F. ) ;
#19558=CARTESIAN_POINT ( 'NONE',  ( -200.0000000000000000, -52.49999999999992895, -52.49999999999999289 ) ) ;
#19566=EDGE_CURVE ( 'NONE', #287, #16217, #3892, .T. ) ;
#19581=ORIENTED_EDGE ( 'NONE', *, *, #24913, .F. ) ;
#19586=CIRCLE ( 'NONE', #8562, 5.000000000000004441 ) ;
#19588=VERTEX_POINT ( 'NONE', #11722 ) ;
#19659=DIRECTION ( 'NONE',  ( 0.000000000000000000, -1.000000000000000000, 0.000000000000000000 ) ) ;
#19709=ORIENTED_EDGE ( 'NONE', *, *, #22794, .T. ) ;
#19719=EDGE_CURVE ( 'NONE', #22425, #8430, #25566, .T. ) ;
#19722=DIRECTION ( 'NONE',  ( -1.000000000000000000, -1.836970198721030181E-16, -0.000000000000000000 ) ) ;
#19733=CARTESIAN_POINT ( 'NONE',  ( 190.0000000000000000, -52.49999999999992895, -52.49999999999999289 ) ) ;
#19742=ORIENTED_EDGE ( 'NONE', *, *, #3862, .F. ) ;
#19768=VECTOR ( 'NONE', #6850, 1000.000000000000000 ) ;
#19780=EDGE_CURVE ( 'NONE', #18643, #15543, #11103, .T. ) ;
#19806=EDGE_LOOP ( 'NONE', ( #17577, #21518 ) ) ;
#19814=CYLINDRICAL_SURFACE ( 'NONE', #1364, 5.000000000000004441 ) ;
#19817=AXIS2_PLACEMENT_3D ( 'NONE', #21730, #1134, #15088 ) ;
#19885=DIRECTION ( 'NONE',  ( 0.000000000000000000, 1.000000000000000000, 0.000000000000000000 ) ) ;
#19901=FACE_BOUND ( 'NONE', #11270, .T. ) ;
#19910=LINE ( 'NONE', #16044, #18434 ) ;
#19917=AXIS2_PLACEMENT_3D ( 'NONE', #6423, #22933, #13206 ) ;
#19936=VERTEX_POINT ( 'NONE', #17841 ) ;
#19937=VERTEX_POINT ( 'NONE', #22121 ) ;
#19963=CIRCLE ( 'NONE', #5952, 5.000000000000004441 ) ;
#19992=LINE ( 'NONE', #4043, #24469 ) ;
#19994=DIRECTION ( 'NONE',  ( 0.000000000000000000, 1.000000000000000000, 0.000000000000000000 ) ) ;
#20024=EDGE_CURVE ( 'NONE', #24679, #433, #22522, .T. ) ;
#20025=DIRECTION ( 'NONE',  ( 1.000000000000000000, 1.836970198721030181E-16, 0.000000000000000000 ) ) ;
#20039=CYLINDRICAL_SURFACE ( 'NONE', #15113, 29.99999999999999645 ) ;
#20077=DIRECTION ( 'NONE',  ( 0.000000000000000000, 1.000000000000000000, 0.000000000000000000 ) ) ;
#20124=ORIENTED_EDGE ( 'NONE', *, *, #7510, .T. ) ;
#20175=EDGE_LOOP ( 'NONE', ( #8531, #19206, #10965, #14845 ) ) ;
#20214=EDGE_LOOP ( 'NONE', ( #11122, #11430, #12477, #11549 ) ) ;
#20273=AXIS2_PLACEMENT_3D ( 'NONE', #23849, #24126, #13733 ) ;
#20293=DIRECTION ( 'NONE',  ( 1.000000000000000000, 1.836970198721030181E-16, -0.000000000000000000 ) ) ;
#20313=EDGE_LOOP ( 'NONE', ( #8999, #1866, #10737, #17161 ) ) ;
#20349=CIRCLE ( 'NONE', #13119, 5.000000000000004441 ) ;
#20353=CARTESIAN_POINT ( 'NONE',  ( -190.0000000000000000, 52.50000000000007816, 52.49999999999999289 ) ) ;
#20394=CARTESIAN_POINT ( 'NONE',  ( 190.0000000000000000, 52.49999999999987210, -82.49999999999998579 ) ) ;
#20400=AXIS2_PLACEMENT_3D ( 'NONE', #11265, #21264, #23134 ) ;
#20459=CARTESIAN_POINT ( 'NONE',  ( -190.0000000000000000, 66.50000000000009948, 66.50000000000005684 ) ) ;
#20476=EDGE_LOOP ( 'NONE', ( #12423, #17933 ) ) ;
#20481=FACE_OUTER_BOUND ( 'NONE', #12756, .T. ) ;
#20501=DIRECTION ( 'NONE',  ( 0.000000000000000000, -1.000000000000000000, 0.000000000000000000 ) ) ;
#20530=CARTESIAN_POINT ( 'NONE',  ( 190.0000000000000000, -71.50000000000002842, -66.50000000000005684 ) ) ;
#20538=DIRECTION ( 'NONE',  ( 0.000000000000000000, -1.000000000000000000, 0.000000000000000000 ) ) ;
#20553=ORIENTED_EDGE ( 'NONE', *, *, #2831, .F. ) ;
#20587=FACE_BOUND ( 'NONE', #20476, .T. ) ;
#20599=CARTESIAN_POINT ( 'NONE',  ( -190.0000000000000000, 61.50000000000009948, 66.50000000000005684 ) ) ;
#20620=VECTOR ( 'NONE', #17375, 1000.000000000000000 ) ;
#20627=EDGE_CURVE ( 'NONE', #3446, #2384, #15348, .T. ) ;
#20650=EDGE_LOOP ( 'NONE', ( #21684, #19538, #13089, #17300 ) ) ;
#20651=VERTEX_POINT ( 'NONE', #20394 ) ;
#20721=CARTESIAN_POINT ( 'NONE',  ( 200.0000000000000000, -52.49999999999972289, -82.49999999999998579 ) ) ;
#20751=FACE_BOUND ( 'NONE', #12858, .T. ) ;
#20761=CARTESIAN_POINT ( 'NONE',  ( 190.0000000000000284, -82.49999999999991473, -52.49999999999977973 ) ) ;
#20798=ADVANCED_FACE ( 'NONE', ( #11512, #19901, #9273, #1685, #13387, #5664 ), #25772, .F. ) ;
#20804=VECTOR ( 'NONE', #17488, 1000.000000000000000 ) ;
#20829=DIRECTION ( 'NONE',  ( 0.000000000000000000, 1.000000000000000000, 0.000000000000000000 ) ) ;
#20847=VERTEX_POINT ( 'NONE', #26041 ) ;
#20868=CARTESIAN_POINT ( 'NONE',  ( -190.0000000000000000, -66.50000000000001421, 66.50000000000005684 ) ) ;
#20874=VECTOR ( 'NONE', #2487, 1000.000000000000000 ) ;
#20917=ORIENTED_EDGE ( 'NONE', *, *, #24526, .T. ) ;
#20931=FACE_OUTER_BOUND ( 'NONE', #1214, .T. ) ;
#20957=CARTESIAN_POINT ( 'NONE',  ( -200.0000000000000000, 74.99999999999995737, 9.184850993605144000E-15 ) ) ;
#21002=ORIENTED_EDGE ( 'NONE', *, *, #17510, .F. ) ;
#21016=ADVANCED_FACE ( 'NONE', ( #16525 ), #6152, .T. ) ;
#21020=CARTESIAN_POINT ( 'NONE',  ( -190.0000000000000000, 1.836970198721033928E-15, 0.000000000000000000 ) ) ;
#21023=DIRECTION ( 'NONE',  ( 1.000000000000000000, 1.836970198721030181E-16, 0.000000000000000000 ) ) ;
#21058=AXIS2_PLACEMENT_3D ( 'NONE', #7994, #22, #15977 ) ;
#21060=CARTESIAN_POINT ( 'NONE',  ( 189.9999999999999716, 82.50000000000008527, -52.49999999999977973 ) ) ;
#21087=DIRECTION ( 'NONE',  ( 1.000000000000000000, -1.836970198721030181E-16, -0.000000000000000000 ) ) ;
#21115=AXIS2_PLACEMENT_3D ( 'NONE', #8037, #3797, #1669 ) ;
#21128=EDGE_CURVE ( 'NONE', #7186, #19106, #23181, .T. ) ;
#21181=ORIENTED_EDGE ( 'NONE', *, *, #22319, .T. ) ;
#21182=VERTEX_POINT ( 'NONE', #10944 ) ;
#21184=DIRECTION ( 'NONE',  ( 1.000000000000000000, 1.836970198721030181E-16, 0.000000000000000000 ) ) ;
#21198=VECTOR ( 'NONE', #11567, 1000.000000000000000 ) ;
#21226=DIRECTION ( 'NONE',  ( 1.000000000000000000, 1.836970198721030181E-16, 0.000000000000000000 ) ) ;
#21234=DIRECTION ( 'NONE',  ( 0.000000000000000000, -1.000000000000000000, 0.000000000000000000 ) ) ;
#21241=AXIS2_PLACEMENT_3D ( 'NONE', #2415, #12382, #10664 ) ;
#21252=DIRECTION ( 'NONE',  ( 0.000000000000000000, 1.000000000000000000, 0.000000000000000000 ) ) ;
#21264=DIRECTION ( 'NONE',  ( -1.000000000000000000, -1.836970198721030181E-16, -0.000000000000000000 ) ) ;
#21273=AXIS2_PLACEMENT_3D ( 'NONE', #13694, #11561, #11693 ) ;
#21274=ADVANCED_FACE ( 'NONE', ( #11186 ), #19814, .F. ) ;
#21283=DIRECTION ( 'NONE',  ( 1.000000000000000000, -1.836970198721030181E-16, -0.000000000000000000 ) ) ;
#21291=FACE_OUTER_BOUND ( 'NONE', #20175, .T. ) ;
#21376=DIRECTION ( 'NONE',  ( 1.000000000000000000, 1.836970198721030181E-16, 0.000000000000000000 ) ) ;
#21394=ORIENTED_EDGE ( 'NONE', *, *, #8145, .T. ) ;
#21411=CARTESIAN_POINT ( 'NONE',  ( -200.0000000000000000, 52.50000000000007816, 52.49999999999999289 ) ) ;
#21418=VERTEX_POINT ( 'NONE', #17809 ) ;
#21491=VECTOR ( 'NONE', #21376, 1000.000000000000000 ) ;
#21518=ORIENTED_EDGE ( 'NONE', *, *, #19719, .T. ) ;
#21523=ORIENTED_EDGE ( 'NONE', *, *, #23949, .T. ) ;
#21527=EDGE_CURVE ( 'NONE', #8430, #22425, #13646, .T. ) ;
#21545=CARTESIAN_POINT ( 'NONE',  ( 200.0000000000000000, -52.49999999999991473, 52.49999999999999289 ) ) ;
#21558=DIRECTION ( 'NONE',  ( 0.000000000000000000, -1.000000000000000000, 0.000000000000000000 ) ) ;
#21578=LINE ( 'NONE', #7089, #8748 ) ;
#21589=ORIENTED_EDGE ( 'NONE', *, *, #25263, .F. ) ;
#21600=CARTESIAN_POINT ( 'NONE',  ( -189.9999999999999716, 82.50000000000008527, 52.49999999999977973 ) ) ;
#21618=CARTESIAN_POINT ( 'NONE',  ( -200.0000000000000000, -69.99999999999995737, 0.000000000000000000 ) ) ;
#21673=CARTESIAN_POINT ( 'NONE',  ( -190.0000000000000000, 74.99999999999995737, 9.184850993605144000E-15 ) ) ;
#21684=ORIENTED_EDGE ( 'NONE', *, *, #2672, .T. ) ;
#21688=FACE_OUTER_BOUND ( 'NONE', #16781, .T. ) ;
#21725=CYLINDRICAL_SURFACE ( 'NONE', #17359, 69.99999999999995737 ) ;
#21730=CARTESIAN_POINT ( 'NONE',  ( -200.0000000000000000, -52.49999999999991473, 52.49999999999999289 ) ) ;
#21753=CARTESIAN_POINT ( 'NONE',  ( -190.0000000000000000, 61.50000000000009948, 66.50000000000005684 ) ) ;
#21808=ORIENTED_EDGE ( 'NONE', *, *, #13301, .F. ) ;
#21811=ADVANCED_FACE ( 'NONE', ( #12097 ), #24212, .F. ) ;
#21822=EDGE_CURVE ( 'NONE', #16552, #24210, #14091, .T. ) ;
#21845=ORIENTED_EDGE ( 'NONE', *, *, #13214, .T. ) ;
#21855=EDGE_CURVE ( 'NONE', #5488, #21418, #6245, .T. ) ;
#21901=AXIS2_PLACEMENT_3D ( 'NONE', #6968, #21087, #2735 ) ;
#21903=VECTOR ( 'NONE', #4020, 1000.000000000000000 ) ;
#21914=AXIS2_PLACEMENT_3D ( 'NONE', #19558, #9576, #26096 ) ;
#21918=EDGE_CURVE ( 'NONE', #19515, #60, #9838, .T. ) ;
#21936=CARTESIAN_POINT ( 'NONE',  ( -190.0000000000000000, -52.49999999999972289, -82.49999999999998579 ) ) ;
#21941=VECTOR ( 'NONE', #25634, 1000.000000000000000 ) ;
#21946=DIRECTION ( 'NONE',  ( 1.000000000000000000, 1.836970198721030181E-16, 0.000000000000000000 ) ) ;
#21953=CIRCLE ( 'NONE', #7485, 5.000000000000004441 ) ;
#21957=CARTESIAN_POINT ( 'NONE',  ( 190.0000000000000284, -82.49999999999991473, -52.49999999999977973 ) ) ;
#21999=CARTESIAN_POINT ( 'NONE',  ( -190.0000000000000000, -52.49999999999970868, 82.49999999999998579 ) ) ;
#22057=CIRCLE ( 'NONE', #4222, 69.99999999999992895 ) ;
#22119=VERTEX_POINT ( 'NONE', #2923 ) ;
#22121=CARTESIAN_POINT ( 'NONE',  ( -200.0000000000000000, 82.50000000000008527, 52.49999999999979394 ) ) ;
#22123=ORIENTED_EDGE ( 'NONE', *, *, #5254, .T. ) ;
#22124=ORIENTED_EDGE ( 'NONE', *, *, #2841, .F. ) ;
#22143=DIRECTION ( 'NONE',  ( -1.000000000000000000, -1.836970198721030181E-16, 0.000000000000000000 ) ) ;
#22144=AXIS2_PLACEMENT_3D ( 'NONE', #19283, #1066, #9884 ) ;
#22162=CARTESIAN_POINT ( 'NONE',  ( 190.0000000000000000, -66.50000000000001421, -66.50000000000005684 ) ) ;
#22166=EDGE_CURVE ( 'NONE', #11718, #14180, #26330, .T. ) ;
#22219=PLANE ( 'NONE',  #17670 ) ;
#22256=EDGE_CURVE ( 'NONE', #20847, #8430, #6994, .T. ) ;
#22270=CARTESIAN_POINT ( 'NONE',  ( 200.0000000000000000, 66.50000000000009948, 66.50000000000005684 ) ) ;
#22319=EDGE_CURVE ( 'NONE', #1888, #24643, #23321, .T. ) ;
#22358=CIRCLE ( 'NONE', #7458, 5.000000000000004441 ) ;
#22384=ORIENTED_EDGE ( 'NONE', *, *, #18249, .T. ) ;
#22398=ORIENTED_EDGE ( 'NONE', *, *, #3689, .T. ) ;
#22425=VERTEX_POINT ( 'NONE', #3097 ) ;
#22483=PLANE ( 'NONE',  #4970 ) ;
#22506=DIRECTION ( 'NONE',  ( -1.000000000000000000, 1.836970198721030181E-16, 0.000000000000000000 ) ) ;
#22515=CARTESIAN_POINT ( 'NONE',  ( -190.0000000000000000, -52.49999999999972289, -82.49999999999998579 ) ) ;
#22518=( NAMED_UNIT ( * ) SI_UNIT ( $, .STERADIAN. ) SOLID_ANGLE_UNIT ( ) );
#22519=EDGE_LOOP ( 'NONE', ( #8432, #3903 ) ) ;
#22522=LINE ( 'NONE', #26262, #12362 ) ;
#22534=LINE ( 'NONE', #20530, #9188 ) ;
#22586=AXIS2_PLACEMENT_3D ( 'NONE', #12277, #10286, #19994 ) ;
#22628=LINE ( 'NONE', #12497, #7030 ) ;
#22649=DIRECTION ( 'NONE',  ( 0.000000000000000000, 1.000000000000000000, 0.000000000000000000 ) ) ;
#22769=DIRECTION ( 'NONE',  ( 0.000000000000000000, -1.000000000000000000, 0.000000000000000000 ) ) ;
#22781=AXIS2_PLACEMENT_3D ( 'NONE', #11850, #13976, #1489 ) ;
#22794=EDGE_CURVE ( 'NONE', #24345, #8862, #16106, .T. ) ;
#22795=DIRECTION ( 'NONE',  ( 1.000000000000000000, 1.836970198721030181E-16, -0.000000000000000000 ) ) ;
#22828=LINE ( 'NONE', #4605, #6225 ) ;
#22848=ORIENTED_EDGE ( 'NONE', *, *, #21822, .T. ) ;
#22855=CARTESIAN_POINT ( 'NONE',  ( -190.0000000000000000, 66.50000000000009948, 66.50000000000005684 ) ) ;
#22876=EDGE_LOOP ( 'NONE', ( #24068, #4594 ) ) ;
#22930=CIRCLE ( 'NONE', #15311, 29.99999999999999289 ) ;
#22933=DIRECTION ( 'NONE',  ( 1.000000000000000000, -1.836970198721030181E-16, -0.000000000000000000 ) ) ;
#22950=CARTESIAN_POINT ( 'NONE',  ( -200.0000000000000000, 0.000000000000000000, 0.000000000000000000 ) ) ;
#23044=DIRECTION ( 'NONE',  ( -1.000000000000000000, 1.836970198721030181E-16, 0.000000000000000000 ) ) ;
#23049=VERTEX_POINT ( 'NONE', #19184 ) ;
#23050=EDGE_LOOP ( 'NONE', ( #9769, #23972 ) ) ;
#23062=DIRECTION ( 'NONE',  ( 1.000000000000000000, 1.836970198721030181E-16, 0.000000000000000000 ) ) ;
#23067=CIRCLE ( 'NONE', #11550, 5.000000000000004441 ) ;
#23068=DIRECTION ( 'NONE',  ( 1.000000000000000000, 1.836970198721030181E-16, 0.000000000000000000 ) ) ;
#23091=FACE_OUTER_BOUND ( 'NONE', #26264, .T. ) ;
#23111=ORIENTED_EDGE ( 'NONE', *, *, #5075, .T. ) ;
#23122=CARTESIAN_POINT ( 'NONE',  ( 190.0000000000000000, -52.49999999999992895, -52.49999999999999289 ) ) ;
#23134=DIRECTION ( 'NONE',  ( 0.000000000000000000, -1.000000000000000000, 0.000000000000000000 ) ) ;
#23166=ADVANCED_FACE ( 'NONE', ( #21688 ), #25691, .F. ) ;
#23174=ORIENTED_EDGE ( 'NONE', *, *, #22319, .F. ) ;
#23181=LINE ( 'NONE', #2562, #509 ) ;
#23186=FACE_BOUND ( 'NONE', #19806, .T. ) ;
#23188=AXIS2_PLACEMENT_3D ( 'NONE', #12260, #17970, #26258 ) ;
#23211=VECTOR ( 'NONE', #17188, 1000.000000000000000 ) ;
#23306=EDGE_CURVE ( 'NONE', #14180, #11718, #16163, .T. ) ;
#23316=EDGE_CURVE ( 'NONE', #13098, #7186, #1250, .T. ) ;
#23321=LINE ( 'NONE', #17317, #13978 ) ;
#23334=CARTESIAN_POINT ( 'NONE',  ( 200.0000000000000000, -52.49999999999970868, 82.49999999999998579 ) ) ;
#23346=AXIS2_PLACEMENT_3D ( 'NONE', #23570, #17321, #3100 ) ;
#23355=DIRECTION ( 'NONE',  ( 1.000000000000000000, 1.836970198721030181E-16, 0.000000000000000000 ) ) ;
#23365=VECTOR ( 'NONE', #3036, 1000.000000000000000 ) ;
#23392=ORIENTED_EDGE ( 'NONE', *, *, #22256, .F. ) ;
#23402=EDGE_CURVE ( 'NONE', #555, #5488, #22930, .T. ) ;
#23414=CIRCLE ( 'NONE', #15744, 5.000000000000004441 ) ;
#23447=CYLINDRICAL_SURFACE ( 'NONE', #23346, 5.000000000000004441 ) ;
#23457=CYLINDRICAL_SURFACE ( 'NONE', #10309, 5.000000000000004441 ) ;
#23519=ORIENTED_EDGE ( 'NONE', *, *, #7750, .T. ) ;
#23538=ADVANCED_FACE ( 'NONE', ( #9336 ), #23447, .F. ) ;
#23552=VERTEX_POINT ( 'NONE', #17958 ) ;
#23569=LINE ( 'NONE', #1099, #6844 ) ;
#23570=CARTESIAN_POINT ( 'NONE',  ( 190.0000000000000000, 66.50000000000009948, -66.50000000000005684 ) ) ;
#23576=ORIENTED_EDGE ( 'NONE', *, *, #3862, .T. ) ;
#23595=PLANE ( 'NONE',  #16428 ) ;
#23598=LINE ( 'NONE', #9889, #25879 ) ;
#23652=AXIS2_PLACEMENT_3D ( 'NONE', #11351, #21226, #19468 ) ;
#23662=DIRECTION ( 'NONE',  ( 0.000000000000000000, 1.000000000000000000, 0.000000000000000000 ) ) ;
#23678=DIRECTION ( 'NONE',  ( 0.000000000000000000, -1.000000000000000000, 0.000000000000000000 ) ) ;
#23713=EDGE_CURVE ( 'NONE', #16552, #19937, #1982, .T. ) ;
#23719=FACE_OUTER_BOUND ( 'NONE', #24338, .T. ) ;
#23752=AXIS2_PLACEMENT_3D ( 'NONE', #20868, #10757, #9274 ) ;
#23754=DIRECTION ( 'NONE',  ( -1.836970198721030181E-16, 1.000000000000000000, 0.000000000000000000 ) ) ;
#23755=ADVANCED_FACE ( 'NONE', ( #24336 ), #3443, .T. ) ;
#23788=LINE ( 'NONE', #1851, #16450 ) ;
#23802=VERTEX_POINT ( 'NONE', #16871 ) ;
#23831=VERTEX_POINT ( 'NONE', #20599 ) ;
#23849=CARTESIAN_POINT ( 'NONE',  ( -190.0000000000000000, -66.50000000000001421, 66.50000000000005684 ) ) ;
#23852=CARTESIAN_POINT ( 'NONE',  ( 200.0000000000000000, 7.347880794884121511E-14, 0.000000000000000000 ) ) ;
#23863=EDGE_CURVE ( 'NONE', #6828, #287, #5495, .T. ) ;
#23903=EDGE_CURVE ( 'NONE', #23932, #16552, #5283, .T. ) ;
#23908=CARTESIAN_POINT ( 'NONE',  ( 190.0000000000000000, 52.50000000000007816, -52.49999999999999289 ) ) ;
#23932=VERTEX_POINT ( 'NONE', #1172 ) ;
#23949=EDGE_CURVE ( 'NONE', #17205, #23049, #8473, .T. ) ;
#23972=ORIENTED_EDGE ( 'NONE', *, *, #5719, .T. ) ;
#23973=PRODUCT_DEFINITION_SHAPE ( 'NONE', 'NONE',  #1112 ) ;
#23997=ORIENTED_EDGE ( 'NONE', *, *, #19220, .F. ) ;
#24003=AXIS2_PLACEMENT_3D ( 'NONE', #14543, #317, #4446 ) ;
#24037=DIRECTION ( 'NONE',  ( -1.000000000000000000, 1.836970198721030181E-16, 0.000000000000000000 ) ) ;
#24068=ORIENTED_EDGE ( 'NONE', *, *, #11594, .T. ) ;
#24106=CARTESIAN_POINT ( 'NONE',  ( 190.0000000000000000, 82.50000000000008527, 52.49999999999979394 ) ) ;
#24117=EDGE_CURVE ( 'NONE', #24643, #17972, #25496, .T. ) ;
#24119=CARTESIAN_POINT ( 'NONE',  ( 200.0000000000000000, 52.50000000000007816, -52.49999999999999289 ) ) ;
#24126=DIRECTION ( 'NONE',  ( -1.000000000000000000, 1.836970198721030181E-16, 0.000000000000000000 ) ) ;
#24140=ORIENTED_EDGE ( 'NONE', *, *, #7750, .F. ) ;
#24142=DIRECTION ( 'NONE',  ( 1.000000000000000000, 1.836970198721030181E-16, 0.000000000000000000 ) ) ;
#24172=EDGE_LOOP ( 'NONE', ( #25470, #21845 ) ) ;
#24181=FACE_OUTER_BOUND ( 'NONE', #16947, .T. ) ;
#24205=ORIENTED_EDGE ( 'NONE', *, *, #17515, .T. ) ;
#24210=VERTEX_POINT ( 'NONE', #19479 ) ;
#24212=CYLINDRICAL_SURFACE ( 'NONE', #2643, 5.000000000000004441 ) ;
#24249=EDGE_LOOP ( 'NONE', ( #118, #14050, #14381, #2421 ) ) ;
#24258=CARTESIAN_POINT ( 'NONE',  ( 190.0000000000000000, 61.50000000000009948, -66.50000000000005684 ) ) ;
#24276=AXIS2_PLACEMENT_3D ( 'NONE', #2249, #14211, #24739 ) ;
#24288=CARTESIAN_POINT ( 'NONE',  ( 190.0000000000000000, 66.50000000000009948, 66.50000000000005684 ) ) ;
#24309=AXIS2_PLACEMENT_3D ( 'NONE', #20353, #2129, #10237 ) ;
#24325=FACE_OUTER_BOUND ( 'NONE', #5747, .T. ) ;
#24336=FACE_OUTER_BOUND ( 'NONE', #12690, .T. ) ;
#24338=EDGE_LOOP ( 'NONE', ( #5884, #1725, #281, #563 ) ) ;
#24345=VERTEX_POINT ( 'NONE', #25621 ) ;
#24350=DIRECTION ( 'NONE',  ( -1.000000000000000000, 1.836970198721030181E-16, 0.000000000000000000 ) ) ;
#24379=ORIENTED_EDGE ( 'NONE', *, *, #3532, .T. ) ;
#24384=ORIENTED_EDGE ( 'NONE', *, *, #21822, .F. ) ;
#24394=DIRECTION ( 'NONE',  ( 0.000000000000000000, 1.000000000000000000, 0.000000000000000000 ) ) ;
#24412=ORIENTED_EDGE ( 'NONE', *, *, #8335, .F. ) ;
#24438=EDGE_CURVE ( 'NONE', #6965, #19453, #10130, .T. ) ;
#24456=STYLED_ITEM('',(#26409),#8871);
#24469=VECTOR ( 'NONE', #7738, 1000.000000000000000 ) ;
#24490=CIRCLE ( 'NONE', #25758, 29.99999999999999645 ) ;
#24503=AXIS2_PLACEMENT_3D ( 'NONE', #659, #10363, #16612 ) ;
#24519=ORIENTED_EDGE ( 'NONE', *, *, #3774, .T. ) ;
#24526=EDGE_CURVE ( 'NONE', #17301, #13098, #3890, .T. ) ;
#24555=DIRECTION ( 'NONE',  ( 1.000000000000000000, 1.836970198721030181E-16, 0.000000000000000000 ) ) ;
#24628=CARTESIAN_POINT ( 'NONE',  ( -190.0000000000000000, -52.49999999999991473, 52.49999999999999289 ) ) ;
#24643=VERTEX_POINT ( 'NONE', #283 ) ;
#24679=VERTEX_POINT ( 'NONE', #25171 ) ;
#24702=ADVANCED_FACE ( 'NONE', ( #820 ), #10797, .T. ) ;
#24739=DIRECTION ( 'NONE',  ( 0.000000000000000000, 1.000000000000000000, 0.000000000000000000 ) ) ;
#24755=EDGE_CURVE ( 'NONE', #6305, #1888, #18502, .T. ) ;
#24814=ORIENTED_EDGE ( 'NONE', *, *, #15794, .T. ) ;
#24852=CARTESIAN_POINT ( 'NONE',  ( 190.0000000000000000, -52.49999999999970868, 82.49999999999998579 ) ) ;
#24865=PRODUCT ( 'Discharge flange', 'Discharge flange', '', ( #17932 ) ) ;
#24883=AXIS2_PLACEMENT_3D ( 'NONE', #22950, #1127, #8843 ) ;
#24901=EDGE_LOOP ( 'NONE', ( #9191, #24379, #163, #10234 ) ) ;
#24909=EDGE_LOOP ( 'NONE', ( #24140, #7429, #4694, #11517 ) ) ;
#24913=EDGE_CURVE ( 'NONE', #7180, #12655, #8054, .T. ) ;
#24918=ORIENTED_EDGE ( 'NONE', *, *, #24438, .T. ) ;
#24943=DIRECTION ( 'NONE',  ( -1.000000000000000000, 0.000000000000000000, -0.000000000000000000 ) ) ;
#24945=AXIS2_PLACEMENT_3D ( 'NONE', #16720, #4632, #14855 ) ;
#24949=ORIENTED_EDGE ( 'NONE', *, *, #10297, .T. ) ;
#25005=DIRECTION ( 'NONE',  ( 0.000000000000000000, -1.000000000000000000, 0.000000000000000000 ) ) ;
#25011=ORIENTED_EDGE ( 'NONE', *, *, #6156, .T. ) ;
#25044=CARTESIAN_POINT ( 'NONE',  ( -190.0000000000000000, -66.50000000000001421, 66.50000000000005684 ) ) ;
#25047=EDGE_LOOP ( 'NONE', ( #9436, #6668, #8896, #23392 ) ) ;
#25050=ORIENTED_EDGE ( 'NONE', *, *, #21855, .T. ) ;
#25058=CARTESIAN_POINT ( 'NONE',  ( 190.0000000000000000, -61.50000000000001421, 66.50000000000005684 ) ) ;
#25085=CYLINDRICAL_SURFACE ( 'NONE', #5325, 5.000000000000004441 ) ;
#25101=CARTESIAN_POINT ( 'NONE',  ( 190.0000000000000000, -52.49999999999972289, -82.49999999999998579 ) ) ;
#25111=ORIENTED_EDGE ( 'NONE', *, *, #14339, .T. ) ;
#25145=DIRECTION ( 'NONE',  ( 1.000000000000000000, -1.836970198721030181E-16, -0.000000000000000000 ) ) ;
#25155=DIRECTION ( 'NONE',  ( -1.000000000000000000, 1.836970198721030181E-16, 0.000000000000000000 ) ) ;
#25168=ORIENTED_EDGE ( 'NONE', *, *, #2256, .F. ) ;
#25171=CARTESIAN_POINT ( 'NONE',  ( 189.9999999999999716, 82.50000000000008527, -52.49999999999977973 ) ) ;
#25181=ORIENTED_EDGE ( 'NONE', *, *, #24438, .F. ) ;
#25215=ORIENTED_EDGE ( 'NONE', *, *, #18249, .F. ) ;
#25229=CARTESIAN_POINT ( 'NONE',  ( 200.0000000000000000, 7.347880794884121511E-14, 0.000000000000000000 ) ) ;
#25253=DIRECTION ( 'NONE',  ( -1.000000000000000000, 1.836970198721030181E-16, 0.000000000000000000 ) ) ;
#25263=EDGE_CURVE ( 'NONE', #11173, #2989, #13594, .T. ) ;
#25316=FACE_BOUND ( 'NONE', #15771, .T. ) ;
#25318=AXIS2_PLACEMENT_3D ( 'NONE', #12543, #16937, #24943 ) ;
#25329=CIRCLE ( 'NONE', #17231, 5.000000000000004441 ) ;
#25333=ORIENTED_EDGE ( 'NONE', *, *, #2014, .F. ) ;
#25335=FACE_OUTER_BOUND ( 'NONE', #2166, .T. ) ;
#25374=CIRCLE ( 'NONE', #19817, 29.99999999999999289 ) ;
#25450=EDGE_CURVE ( 'NONE', #24210, #555, #9345, .T. ) ;
#25470=ORIENTED_EDGE ( 'NONE', *, *, #11900, .T. ) ;
#25496=CIRCLE ( 'NONE', #6794, 30.00000000000000355 ) ;
#25550=CARTESIAN_POINT ( 'NONE',  ( 190.0000000000000000, -66.50000000000001421, 66.50000000000005684 ) ) ;
#25566=CIRCLE ( 'NONE', #5165, 5.000000000000004441 ) ;
#25600=ORIENTED_EDGE ( 'NONE', *, *, #12384, .T. ) ;
#25621=CARTESIAN_POINT ( 'NONE',  ( -190.0000000000000000, -61.50000000000001421, -66.50000000000005684 ) ) ;
#25628=FACE_OUTER_BOUND ( 'NONE', #2120, .T. ) ;
#25634=DIRECTION ( 'NONE',  ( 1.000000000000000000, 1.836970198721030181E-16, 0.000000000000000000 ) ) ;
#25639=CARTESIAN_POINT ( 'NONE',  ( -200.0000000000000000, -52.49999999999972289, -82.49999999999998579 ) ) ;
#25673=FACE_OUTER_BOUND ( 'NONE', #7692, .T. ) ;
#25682=ORIENTED_EDGE ( 'NONE', *, *, #6869, .F. ) ;
#25687=EDGE_LOOP ( 'NONE', ( #8200, #19709, #10102, #10276 ) ) ;
#25691=CYLINDRICAL_SURFACE ( 'NONE', #12717, 69.99999999999995737 ) ;
#25709=DIRECTION ( 'NONE',  ( 1.000000000000000000, 1.836970198721030181E-16, 0.000000000000000000 ) ) ;
#25712=CARTESIAN_POINT ( 'NONE',  ( 200.0000000000000000, 61.50000000000009948, -66.50000000000005684 ) ) ;
#25719=ORIENTED_EDGE ( 'NONE', *, *, #10443, .T. ) ;
#25722=CARTESIAN_POINT ( 'NONE',  ( -190.0000000000000000, -71.50000000000002842, -66.50000000000005684 ) ) ;
#25740=EDGE_CURVE ( 'NONE', #992, #15670, #19963, .T. ) ;
#25747=FACE_OUTER_BOUND ( 'NONE', #17977, .T. ) ;
#25752=CIRCLE ( 'NONE', #22781, 5.000000000000004441 ) ;
#25754=DIRECTION ( 'NONE',  ( 0.000000000000000000, 1.000000000000000000, 0.000000000000000000 ) ) ;
#25758=AXIS2_PLACEMENT_3D ( 'NONE', #23122, #4895, #21252 ) ;
#25760=CARTESIAN_POINT ( 'NONE',  ( 190.0000000000000000, 71.50000000000009948, -66.50000000000005684 ) ) ;
#25772=PLANE ( 'NONE',  #1313 ) ;
#25789=CARTESIAN_POINT ( 'NONE',  ( -200.0000000000000000, 69.99999999999998579, 8.572527594031466682E-15 ) ) ;
#25868=DIRECTION ( 'NONE',  ( -1.000000000000000000, -1.836970198721030181E-16, -0.000000000000000000 ) ) ;
#25879=VECTOR ( 'NONE', #17992, 1000.000000000000000 ) ;
#25902=FACE_OUTER_BOUND ( 'NONE', #3458, .T. ) ;
#25926=CARTESIAN_POINT ( 'NONE',  ( 190.0000000000000000, -52.49999999999972289, -82.49999999999998579 ) ) ;
#25939=ORIENTED_EDGE ( 'NONE', *, *, #19163, .F. ) ;
#25940=DIRECTION ( 'NONE',  ( 1.000000000000000000, 0.000000000000000000, -0.000000000000000000 ) ) ;
#25946=ORIENTED_EDGE ( 'NONE', *, *, #5254, .F. ) ;
#25957=DIRECTION ( 'NONE',  ( 0.000000000000000000, -1.000000000000000000, 0.000000000000000000 ) ) ;
#25961=DIRECTION ( 'NONE',  ( -1.000000000000000000, 1.836970198721030181E-16, 0.000000000000000000 ) ) ;
#25979=ORIENTED_EDGE ( 'NONE', *, *, #24117, .F. ) ;
#25992=AXIS2_PLACEMENT_3D ( 'NONE', #4576, #18800, #12813 ) ;
#25994=EDGE_LOOP ( 'NONE', ( #23576, #13460, #24384, #10334 ) ) ;
#26022=AXIS2_PLACEMENT_3D ( 'NONE', #21545, #17795, #9826 ) ;
#26041=CARTESIAN_POINT ( 'NONE',  ( -190.0000000000000000, 61.50000000000009948, -66.50000000000005684 ) ) ;
#26081=ORIENTED_EDGE ( 'NONE', *, *, #26327, .T. ) ;
#26087=ORIENTED_EDGE ( 'NONE', *, *, #6380, .F. ) ;
#26096=DIRECTION ( 'NONE',  ( 0.000000000000000000, 1.000000000000000000, 0.000000000000000000 ) ) ;
#26110=CARTESIAN_POINT ( 'NONE',  ( -190.0000000000000000, -71.50000000000002842, -66.50000000000005684 ) ) ;
#26165=ADVANCED_FACE ( 'NONE', ( #1589 ), #15069, .T. ) ;
#26183=AXIS2_PLACEMENT_3D ( 'NONE', #21411, #13290, #19659 ) ;
#26192=VECTOR ( 'NONE', #23062, 1000.000000000000000 ) ;
#26217=CARTESIAN_POINT ( 'NONE',  ( -190.0000000000000000, -61.50000000000001421, 66.50000000000005684 ) ) ;
#26258=DIRECTION ( 'NONE',  ( 0.000000000000000000, -1.000000000000000000, 0.000000000000000000 ) ) ;
#26262=CARTESIAN_POINT ( 'NONE',  ( 189.9999999999999716, 82.50000000000008527, 52.49999999999977973 ) ) ;
#26264=EDGE_LOOP ( 'NONE', ( #15394, #7067, #9186, #9956 ) ) ;
#26310=CARTESIAN_POINT ( 'NONE',  ( 200.0000000000000000, -66.50000000000001421, -66.50000000000005684 ) ) ;
#26317=EDGE_LOOP ( 'NONE', ( #21181, #14605, #11148, #8536 ) ) ;
#26327=EDGE_CURVE ( 'NONE', #23049, #17205, #16368, .T. ) ;
#26330=CIRCLE ( 'NONE', #3792, 5.000000000000004441 ) ;
#26331=DIRECTION ( 'NONE',  ( 1.836970198721030181E-16, -1.000000000000000000, 0.000000000000000000 ) ) ;
#26345=EDGE_LOOP ( 'NONE', ( #25600, #12163 ) ) ;
#26403=COLOUR_RGB('Off White',0.89,0.88,0.83);
#26404=FILL_AREA_STYLE_COLOUR('',#26403);
#26405=FILL_AREA_STYLE('',(#26404));
#26406=SURFACE_STYLE_FILL_AREA(#26405);
#26407=SURFACE_SIDE_STYLE('',(#26406));
#26408=SURFACE_STYLE_USAGE(.BOTH.,#26407);
#26409=PRESENTATION_STYLE_ASSIGNMENT((#26408));
ENDSEC;
END-ISO-10303-21;
